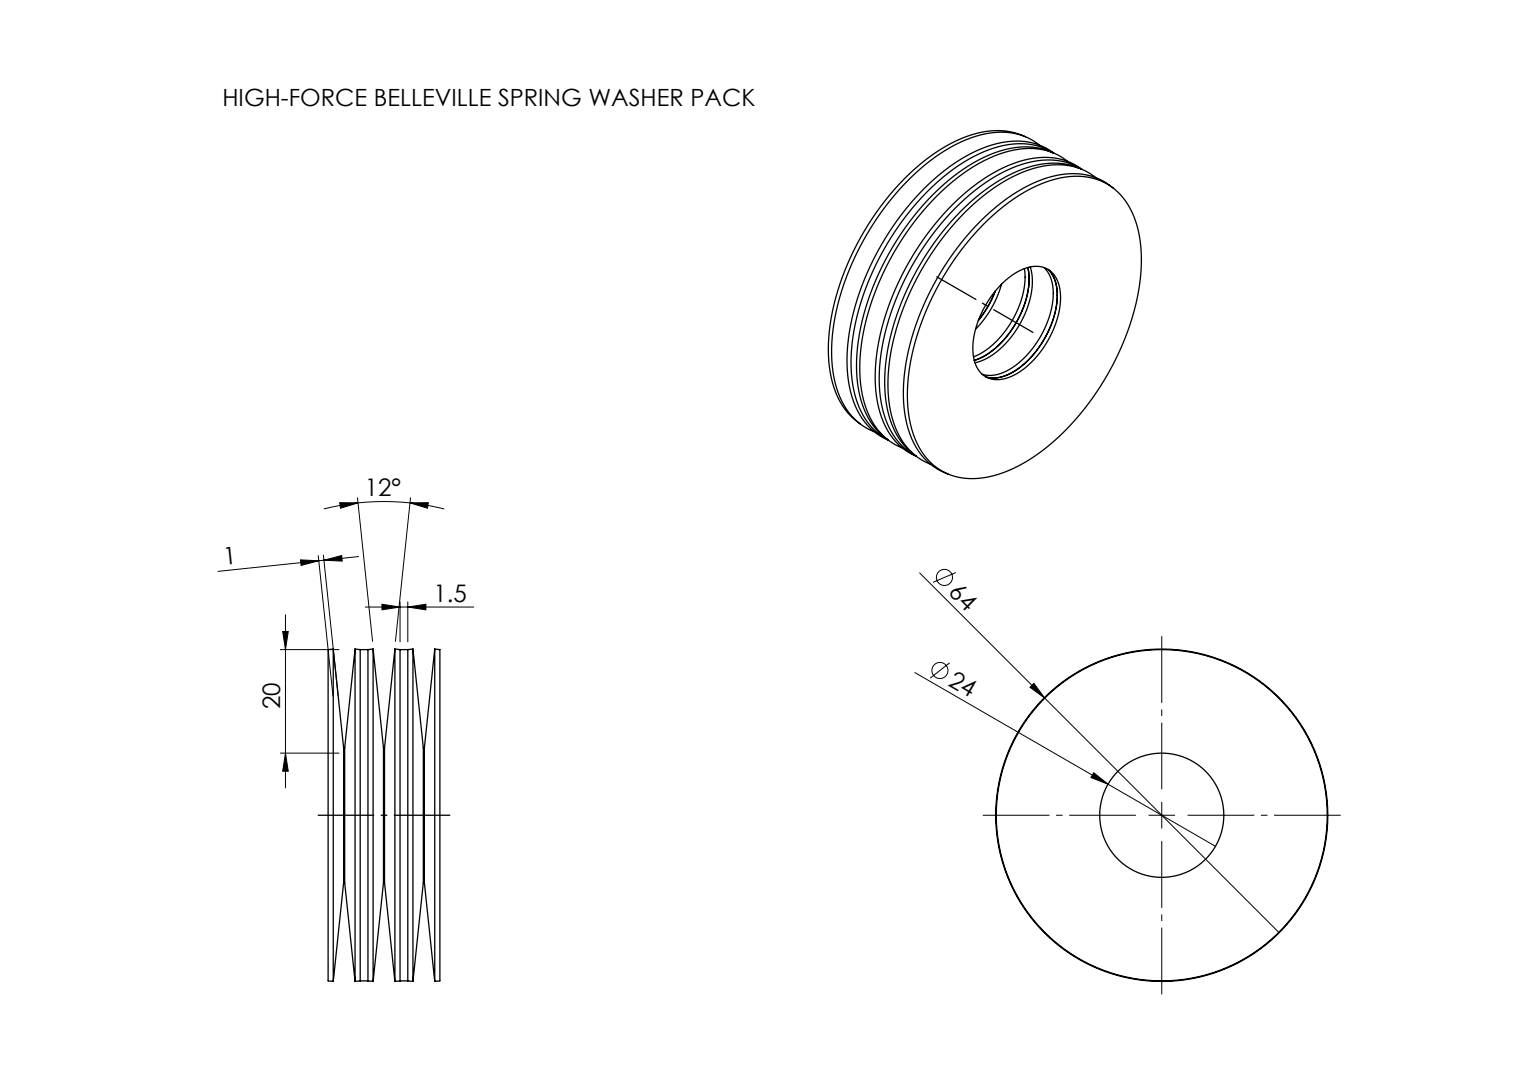
ISO-10303-21;
HEADER;
FILE_DESCRIPTION (('STEP AP214'),
    '1' );
FILE_NAME ('High-Force Belleville Spring Washer Pack.step',
    '2026-10-08T07:58:12',
    ( '' ),
    ( '' ),
    'SwSTEP 2.0',
    'SolidWorks 2026',
    '' );
FILE_SCHEMA (( 'AUTOMOTIVE_DESIGN' ));
ENDSEC;

DATA;
#82=VERTEX_POINT ( 'NONE', #32615 ) ;
#84=EDGE_LOOP ( 'NONE', ( #4042, #16247, #32529, #21714 ) ) ;
#116=ORIENTED_EDGE ( 'NONE', *, *, #1238, .F. ) ;
#123=ORIENTED_EDGE ( 'NONE', *, *, #8294, .T. ) ;
#126=CONICAL_SURFACE ( 'NONE', #19149, 32.00000000000005684, 0.1047197551196217685 ) ;
#134=CARTESIAN_POINT ( 'NONE',  ( 108.1100194822685836, 155.0000000000000000, 0.000000000000000000 ) ) ;
#174=( NAMED_UNIT ( * ) SI_UNIT ( $, .STERADIAN. ) SOLID_ANGLE_UNIT ( ) );
#179=EDGE_CURVE ( 'NONE', #29148, #5220, #18847, .T. ) ;
#189=CARTESIAN_POINT ( 'NONE',  ( 90.49452189536829394, 155.0000000000000000, 0.000000000000000000 ) ) ;
#195=CIRCLE ( 'NONE', #24668, 12.10452846326762177 ) ;
#196=CARTESIAN_POINT ( 'NONE',  ( 93.60208470531338776, 155.0000000000000000, 12.00000000000001066 ) ) ;
#210=VERTEX_POINT ( 'NONE', #17453 ) ;
#228=CIRCLE ( 'NONE', #27934, 13.00000000000001066 ) ;
#244=ORIENTED_EDGE ( 'NONE', *, *, #9158, .T. ) ;
#290=DIRECTION ( 'NONE',  ( 1.000000000000000000, -0.000000000000000000, -0.000000000000000000 ) ) ;
#316=DIRECTION ( 'NONE',  ( 0.000000000000000000, 0.000000000000000000, -1.000000000000000000 ) ) ;
#330=FILL_AREA_STYLE ('',( #26891 ) ) ;
#360=ORIENTED_EDGE ( 'NONE', *, *, #7714, .F. ) ;
#380=DIRECTION ( 'NONE',  ( -1.000000000000000000, 0.000000000000000000, 0.000000000000000000 ) ) ;
#424=DIRECTION ( 'NONE',  ( 0.000000000000000000, 0.000000000000000000, -1.000000000000000000 ) ) ;
#445=ADVANCED_FACE ( 'NONE', ( #32704 ), #17380, .F. ) ;
#456=VECTOR ( 'NONE', #17521, 1000.000000000000227 ) ;
#471=CIRCLE ( 'NONE', #10841, 12.10452846326762177 ) ;
#546=VERTEX_POINT ( 'NONE', #19601 ) ;
#555=LINE ( 'NONE', #10948, #13247 ) ;
#563=CARTESIAN_POINT ( 'NONE',  ( 102.4138169258850581, 155.0000000000000000, 0.000000000000000000 ) ) ;
#611=FACE_OUTER_BOUND ( 'NONE', #24311, .T. ) ;
#622=EDGE_CURVE ( 'NONE', #30802, #33225, #4723, .T. ) ;
#624=EDGE_CURVE ( 'NONE', #17270, #23382, #19967, .T. ) ;
#631=CARTESIAN_POINT ( 'NONE',  ( 100.2066581602377653, 155.0000000000000000, -13.00000000000001066 ) ) ;
#701=AXIS2_PLACEMENT_3D ( 'NONE', #11341, #16437, #6045 ) ;
#707=CARTESIAN_POINT ( 'NONE',  ( 94.70964751525852421, 155.0000000000000000, 32.10452846326766974 ) ) ;
#715=CIRCLE ( 'NONE', #5600, 13.00000000000003908 ) ;
#727=DIRECTION ( 'NONE',  ( 1.000000000000000000, -0.000000000000000000, -0.000000000000000000 ) ) ;
#732=DIRECTION ( 'NONE',  ( 0.000000000000000000, 0.000000000000000000, 1.000000000000000000 ) ) ;
#748=CARTESIAN_POINT ( 'NONE',  ( 100.4058500716420781, 155.0000000000000000, 0.000000000000000000 ) ) ;
#764=ADVANCED_FACE ( 'NONE', ( #27053 ), #13424, .T. ) ;
#767=EDGE_CURVE ( 'NONE', #31501, #25247, #11551, .T. ) ;
#794=CARTESIAN_POINT ( 'NONE',  ( 101.3062541159399075, 155.0000000000000000, -12.00000000000001066 ) ) ;
#824=DIRECTION ( 'NONE',  ( 1.000000000000000000, -0.000000000000000000, -0.000000000000000000 ) ) ;
#849=LINE ( 'NONE', #23689, #23558 ) ;
#881=CONICAL_SURFACE ( 'NONE', #18301, 31.00000000000000000, 1.466076571675255957 ) ;
#885=CARTESIAN_POINT ( 'NONE',  ( 92.70168066101555837, 155.0000000000000000, -13.00000000000003908 ) ) ;
#889=VERTEX_POINT ( 'NONE', #33000 ) ;
#899=ORIENTED_EDGE ( 'NONE', *, *, #32978, .F. ) ;
#910=ORIENTED_EDGE ( 'NONE', *, *, #16888, .T. ) ;
#916=APPLICATION_CONTEXT ( 'automotive_design' ) ;
#931=EDGE_LOOP ( 'NONE', ( #7883, #32623, #17410, #12258 ) ) ;
#954=CARTESIAN_POINT ( 'NONE',  ( 109.0104235265664272, 155.0000000000000000, -11.99999999999998224 ) ) ;
#978=EDGE_CURVE ( 'NONE', #23779, #33225, #14441, .T. ) ;
#984=EDGE_LOOP ( 'NONE', ( #28690, #5687, #6551, #10597 ) ) ;
#1046=CARTESIAN_POINT ( 'NONE',  ( 89.50000000000002842, 155.0000000000000000, 0.000000000000000000 ) ) ;
#1054=EDGE_CURVE ( 'NONE', #14849, #9110, #2180, .T. ) ;
#1085=ORIENTED_EDGE ( 'NONE', *, *, #22443, .T. ) ;
#1106=EDGE_LOOP ( 'NONE', ( #29137, #28238, #18476, #24027 ) ) ;
#1150=VECTOR ( 'NONE', #31313, 1000.000000000000000 ) ;
#1161=ORIENTED_EDGE ( 'NONE', *, *, #624, .T. ) ;
#1186=DIRECTION ( 'NONE',  ( -0.1045284632676468234, 1.217938055844715641E-16, -0.9945218953682740670 ) ) ;
#1204=CIRCLE ( 'NONE', #21871, 32.10452846326769816 ) ;
#1216=DIRECTION ( 'NONE',  ( -0.1045284632676468234, 1.217938055844715641E-16, -0.9945218953682740670 ) ) ;
#1225=LINE ( 'NONE', #11455, #20091 ) ;
#1236=VECTOR ( 'NONE', #1186, 1000.000000000000000 ) ;
#1238=EDGE_CURVE ( 'NONE', #29217, #23382, #10861, .T. ) ;
#1251=AXIS2_PLACEMENT_3D ( 'NONE', #4410, #33022, #24855 ) ;
#1255=CARTESIAN_POINT ( 'NONE',  ( 99.30625411593993590, 155.0000000000000000, 0.000000000000000000 ) ) ;
#1263=AXIS2_PLACEMENT_3D ( 'NONE', #30747, #23072, #15236 ) ;
#1285=( GEOMETRIC_REPRESENTATION_CONTEXT ( 3 ) GLOBAL_UNCERTAINTY_ASSIGNED_CONTEXT ( ( #28742 ) ) GLOBAL_UNIT_ASSIGNED_CONTEXT ( ( #21117, #12788, #28297 ) ) REPRESENTATION_CONTEXT ( 'NONE', 'WORKASPACE' ) );
#1300=LINE ( 'NONE', #25129, #6401 ) ;
#1393=CARTESIAN_POINT ( 'NONE',  ( 103.3032345859876102, 155.0000000000000000, 0.000000000000000000 ) ) ;
#1394=EDGE_CURVE ( 'NONE', #20431, #4805, #4178, .T. ) ;
#1411=EDGE_CURVE ( 'NONE', #11140, #8132, #1300, .T. ) ;
#1412=CARTESIAN_POINT ( 'NONE',  ( 109.0104235265664272, 155.0000000000000000, 0.000000000000000000 ) ) ;
#1482=CONICAL_SURFACE ( 'NONE', #33017, 31.00000000000000000, 1.466076571675244411 ) ;
#1485=CONICAL_SURFACE ( 'NONE', #10213, 32.00000000000002842, 0.1047197551196464710 ) ;
#1493=AXIS2_PLACEMENT_3D ( 'NONE', #20677, #28516, #8228 ) ;
#1518=AXIS2_PLACEMENT_3D ( 'NONE', #2238, #23684, #33580 ) ;
#1519=CARTESIAN_POINT ( 'NONE',  ( 97.20416941062678973, 155.0000000000000000, -32.00000000000000000 ) ) ;
#1564=DIRECTION ( 'NONE',  ( 0.000000000000000000, 0.000000000000000000, -1.000000000000000000 ) ) ;
#1566=EDGE_LOOP ( 'NONE', ( #30199, #32332, #23952, #6736 ) ) ;
#1576=CARTESIAN_POINT ( 'NONE',  ( 92.60208470531341618, 155.0000000000000000, 31.00000000000000000 ) ) ;
#1579=AXIS2_PLACEMENT_3D ( 'NONE', #10338, #33321, #5373 ) ;
#1590=DIRECTION ( 'NONE',  ( 1.000000000000000000, -0.000000000000000000, -0.000000000000000000 ) ) ;
#1605=CONICAL_SURFACE ( 'NONE', #3771, 31.00000000000000000, 1.466076571675244411 ) ;
#1612=DIRECTION ( 'NONE',  ( 0.000000000000000000, 0.000000000000000000, -1.000000000000000000 ) ) ;
#1617=EDGE_LOOP ( 'NONE', ( #31985, #3988, #7749, #18258 ) ) ;
#1622=ORIENTED_EDGE ( 'NONE', *, *, #19447, .F. ) ;
#1694=VERTEX_POINT ( 'NONE', #5033 ) ;
#1705=EDGE_LOOP ( 'NONE', ( #13701, #14443, #3420, #26950 ) ) ;
#1724=CARTESIAN_POINT ( 'NONE',  ( 108.0049454219347354, 155.0000000000000000, 0.000000000000000000 ) ) ;
#1753=ADVANCED_FACE ( 'NONE', ( #12697 ), #31102, .F. ) ;
#1778=CIRCLE ( 'NONE', #1251, 12.00000000000001066 ) ;
#1787=CONICAL_SURFACE ( 'NONE', #24631, 32.10452846326766974, 1.466076571675243523 ) ;
#1802=DIRECTION ( 'NONE',  ( 1.000000000000000000, -0.000000000000000000, -0.000000000000000000 ) ) ;
#1897=DIRECTION ( 'NONE',  ( 0.000000000000000000, 0.000000000000000000, 1.000000000000000000 ) ) ;
#1912=CARTESIAN_POINT ( 'NONE',  ( 100.4058500716420781, 155.0000000000000000, 0.000000000000000000 ) ) ;
#1918=DIRECTION ( 'NONE',  ( 0.000000000000000000, 0.000000000000000000, -1.000000000000000000 ) ) ;
#1975=DIRECTION ( 'NONE',  ( 1.000000000000000000, -0.000000000000000000, -0.000000000000000000 ) ) ;
#1993=DIRECTION ( 'NONE',  ( 0.000000000000000000, 0.000000000000000000, -1.000000000000000000 ) ) ;
#1996=ORIENTED_EDGE ( 'NONE', *, *, #12415, .T. ) ;
#2013=FACE_OUTER_BOUND ( 'NONE', #29654, .T. ) ;
#2018=APPLICATION_CONTEXT ( 'automotive_design' ) ;
#2030=VECTOR ( 'NONE', #31162, 999.9999999999998863 ) ;
#2040=EDGE_CURVE ( 'NONE', #21429, #17270, #21992, .T. ) ;
#2041=DIRECTION ( 'NONE',  ( 1.000000000000000000, -0.000000000000000000, -0.000000000000000000 ) ) ;
#2047=ADVANCED_FACE ( 'NONE', ( #16205 ), #18935, .T. ) ;
#2067=DIRECTION ( 'NONE',  ( 0.000000000000000000, 0.000000000000000000, -1.000000000000000000 ) ) ;
#2074=DIRECTION ( 'NONE',  ( 1.000000000000000000, -0.000000000000000000, -0.000000000000000000 ) ) ;
#2090=CIRCLE ( 'NONE', #13506, 12.10452846326765020 ) ;
#2092=ORIENTED_EDGE ( 'NONE', *, *, #32224, .T. ) ;
#2095=EDGE_CURVE ( 'NONE', #31583, #27125, #471, .T. ) ;
#2103=AXIS2_PLACEMENT_3D ( 'NONE', #21080, #17861, #5416 ) ;
#2126=DIRECTION ( 'NONE',  ( -1.000000000000000000, 0.000000000000000000, 0.000000000000000000 ) ) ;
#2131=VECTOR ( 'NONE', #9268, 1000.000000000000000 ) ;
#2168=CARTESIAN_POINT ( 'NONE',  ( 92.60208470531341618, 155.0000000000000000, -12.10452846326763598 ) ) ;
#2180=LINE ( 'NONE', #2696, #10740 ) ;
#2186=CARTESIAN_POINT ( 'NONE',  ( 92.60208470531341618, 155.0000000000000000, 0.000000000000000000 ) ) ;
#2209=DIRECTION ( 'NONE',  ( 1.000000000000000000, -0.000000000000000000, -0.000000000000000000 ) ) ;
#2210=VERTEX_POINT ( 'NONE', #25054 ) ;
#2238=CARTESIAN_POINT ( 'NONE',  ( 97.20416941062678973, 155.0000000000000000, 0.000000000000000000 ) ) ;
#2248=DIRECTION ( 'NONE',  ( 0.000000000000000000, 0.000000000000000000, -1.000000000000000000 ) ) ;
#2284=AXIS2_PLACEMENT_3D ( 'NONE', #19617, #14669, #2067 ) ;
#2288=LINE ( 'NONE', #12842, #12668 ) ;
#2313=VECTOR ( 'NONE', #14414, 1000.000000000000114 ) ;
#2325=EDGE_CURVE ( 'NONE', #33225, #30802, #15185, .T. ) ;
#2357=DIRECTION ( 'NONE',  ( 1.000000000000000000, -0.000000000000000000, -0.000000000000000000 ) ) ;
#2368=AXIS2_PLACEMENT_3D ( 'NONE', #10280, #31377, #20658 ) ;
#2384=ORIENTED_EDGE ( 'NONE', *, *, #27422, .T. ) ;
#2397=CARTESIAN_POINT ( 'NONE',  ( 92.60208470531341618, 155.0000000000000000, 32.00000000000002842 ) ) ;
#2404=AXIS2_PLACEMENT_3D ( 'NONE', #8872, #11941, #4266 ) ;
#2457=ORIENTED_EDGE ( 'NONE', *, *, #7239, .F. ) ;
#2463=ORIENTED_EDGE ( 'NONE', *, *, #19799, .F. ) ;
#2483=DIRECTION ( 'NONE',  ( 0.000000000000000000, 0.000000000000000000, -1.000000000000000000 ) ) ;
#2490=CARTESIAN_POINT ( 'NONE',  ( 95.70416941062676131, 155.0000000000000000, 0.000000000000000000 ) ) ;
#2495=FACE_OUTER_BOUND ( 'NONE', #5360, .T. ) ;
#2548=CIRCLE ( 'NONE', #16678, 12.00000000000001066 ) ;
#2652=LINE ( 'NONE', #25643, #15958 ) ;
#2659=CARTESIAN_POINT ( 'NONE',  ( 92.60208470531341618, 155.0000000000000000, 12.10452846326765020 ) ) ;
#2696=CARTESIAN_POINT ( 'NONE',  ( 92.60208470531341618, 155.0000000000000000, -12.99999999999999822 ) ) ;
#2730=EDGE_CURVE ( 'NONE', #20904, #29148, #11559, .T. ) ;
#2735=EDGE_CURVE ( 'NONE', #20904, #6439, #27778, .T. ) ;
#2760=VERTEX_POINT ( 'NONE', #11222 ) ;
#2850=DIRECTION ( 'NONE',  ( 1.000000000000000000, -0.000000000000000000, -0.000000000000000000 ) ) ;
#2853=ADVANCED_FACE ( 'NONE', ( #21776 ), #30510, .T. ) ;
#2878=DIRECTION ( 'NONE',  ( 1.000000000000000000, -0.000000000000000000, -0.000000000000000000 ) ) ;
#2879=ORIENTED_EDGE ( 'NONE', *, *, #30577, .F. ) ;
#2942=DIRECTION ( 'NONE',  ( -0.1045284632676468234, 0.000000000000000000, 0.9945218953682740670 ) ) ;
#2962=CARTESIAN_POINT ( 'NONE',  ( 97.30927364589244632, 155.0000000000000000, 0.000000000000000000 ) ) ;
#2963=ORIENTED_EDGE ( 'NONE', *, *, #18143, .F. ) ;
#3002=ORIENTED_EDGE ( 'NONE', *, *, #15223, .F. ) ;
#3028=ADVANCED_FACE ( 'NONE', ( #2013 ), #6784, .F. ) ;
#3080=AXIS2_PLACEMENT_3D ( 'NONE', #20994, #31391, #8061 ) ;
#3117=LINE ( 'NONE', #30021, #19378 ) ;
#3146=VECTOR ( 'NONE', #32555, 1000.000000000000000 ) ;
#3149=EDGE_LOOP ( 'NONE', ( #21685, #21772, #23410, #22654 ) ) ;
#3154=DIRECTION ( 'NONE',  ( 1.000000000000000000, -0.000000000000000000, -0.000000000000000000 ) ) ;
#3157=VERTEX_POINT ( 'NONE', #27733 ) ;
#3188=CARTESIAN_POINT ( 'NONE',  ( 98.19869130599479945, 155.0000000000000000, -32.10452846326769816 ) ) ;
#3207=ORIENTED_EDGE ( 'NONE', *, *, #767, .T. ) ;
#3259=CARTESIAN_POINT ( 'NONE',  ( 92.60208470531341618, 155.0000000000000000, 0.000000000000000000 ) ) ;
#3279=ADVANCED_FACE ( 'NONE', ( #4905 ), #25518, .T. ) ;
#3308=DIRECTION ( 'NONE',  ( -0.9945218953682772867, 1.280104479604772081E-17, -0.1045284632676156678 ) ) ;
#3316=CARTESIAN_POINT ( 'NONE',  ( 100.4058500716420781, 155.0000000000000000, -12.99999999999998401 ) ) ;
#3346=FACE_OUTER_BOUND ( 'NONE', #29316, .T. ) ;
#3358=CONICAL_SURFACE ( 'NONE', #11467, 32.10452846326769816, 1.466076571675243523 ) ;
#3415=VECTOR ( 'NONE', #9617, 1000.000000000000000 ) ;
#3420=ORIENTED_EDGE ( 'NONE', *, *, #23975, .T. ) ;
#3440=CARTESIAN_POINT ( 'NONE',  ( 100.2066581602377653, 155.0000000000000000, 0.000000000000000000 ) ) ;
#3445=EDGE_CURVE ( 'NONE', #889, #23658, #5075, .T. ) ;
#3446=VECTOR ( 'NONE', #9745, 1000.000000000000000 ) ;
#3479=CARTESIAN_POINT ( 'NONE',  ( 92.60208470531341618, 155.0000000000000000, -31.00000000000000000 ) ) ;
#3490=AXIS2_PLACEMENT_3D ( 'NONE', #3890, #6624, #19900 ) ;
#3537=EDGE_CURVE ( 'NONE', #20010, #29148, #19314, .T. ) ;
#3619=ORIENTED_EDGE ( 'NONE', *, *, #23140, .T. ) ;
#3621=AXIS2_PLACEMENT_3D ( 'NONE', #11749, #27088, #9530 ) ;
#3627=DIRECTION ( 'NONE',  ( 0.000000000000000000, 0.000000000000000000, 1.000000000000000000 ) ) ;
#3650=FACE_OUTER_BOUND ( 'NONE', #25283, .T. ) ;
#3652=ORIENTED_EDGE ( 'NONE', *, *, #30577, .T. ) ;
#3660=ORIENTED_EDGE ( 'NONE', *, *, #2325, .T. ) ;
#3661=LINE ( 'NONE', #7590, #25185 ) ;
#3665=CONICAL_SURFACE ( 'NONE', #8043, 31.00000000000000000, 1.466076571675243967 ) ;
#3667=CIRCLE ( 'NONE', #23258, 31.00000000000000000 ) ;
#3670=DIRECTION ( 'NONE',  ( 0.000000000000000000, 0.000000000000000000, -1.000000000000000000 ) ) ;
#3694=VECTOR ( 'NONE', #17304, 1000.000000000000227 ) ;
#3713=CARTESIAN_POINT ( 'NONE',  ( 107.0104235265664556, 155.0000000000000000, -11.99999999999998224 ) ) ;
#3715=DIRECTION ( 'NONE',  ( 0.000000000000000000, 0.000000000000000000, -1.000000000000000000 ) ) ;
#3744=ORIENTED_EDGE ( 'NONE', *, *, #8275, .T. ) ;
#3753=VECTOR ( 'NONE', #32543, 1000.000000000000000 ) ;
#3771=AXIS2_PLACEMENT_3D ( 'NONE', #1393, #29678, #11783 ) ;
#3778=DIRECTION ( 'NONE',  ( 1.000000000000000000, -0.000000000000000000, -0.000000000000000000 ) ) ;
#3786=EDGE_LOOP ( 'NONE', ( #21693, #360, #32034, #18428 ) ) ;
#3805=ORIENTED_EDGE ( 'NONE', *, *, #29067, .T. ) ;
#3869=EDGE_LOOP ( 'NONE', ( #22538, #19080, #7962, #23492 ) ) ;
#3881=CARTESIAN_POINT ( 'NONE',  ( 105.0134430565187387, 155.0000000000000000, 0.000000000000000000 ) ) ;
#3890=CARTESIAN_POINT ( 'NONE',  ( 95.59906517536109050, 155.0000000000000000, 0.000000000000000000 ) ) ;
#3903=ORIENTED_EDGE ( 'NONE', *, *, #15621, .F. ) ;
#3925=CIRCLE ( 'NONE', #14822, 31.00000000000000000 ) ;
#3952=CIRCLE ( 'NONE', #23003, 13.00000000000003908 ) ;
#3977=AXIS2_PLACEMENT_3D ( 'NONE', #10455, #380, #25940 ) ;
#3982=DIRECTION ( 'NONE',  ( 1.000000000000000000, -0.000000000000000000, -0.000000000000000000 ) ) ;
#3988=ORIENTED_EDGE ( 'NONE', *, *, #4099, .T. ) ;
#4004=AXIS2_PLACEMENT_3D ( 'NONE', #13608, #6100, #18734 ) ;
#4006=DIRECTION ( 'NONE',  ( 0.000000000000000000, 0.000000000000000000, -1.000000000000000000 ) ) ;
#4042=ORIENTED_EDGE ( 'NONE', *, *, #11060, .F. ) ;
#4049=AXIS2_PLACEMENT_3D ( 'NONE', #21081, #18855, #13739 ) ;
#4058=EDGE_CURVE ( 'NONE', #19467, #20904, #8066, .T. ) ;
#4093=CARTESIAN_POINT ( 'NONE',  ( 89.50000000000002842, 155.0000000000000000, 32.00000000000002842 ) ) ;
#4099=EDGE_CURVE ( 'NONE', #26344, #8252, #7568, .T. ) ;
#4131=CARTESIAN_POINT ( 'NONE',  ( 93.60208470531338776, 155.0000000000000000, 0.000000000000000000 ) ) ;
#4154=CARTESIAN_POINT ( 'NONE',  ( 97.30927364589244632, 155.0000000000000000, -31.00000000000000000 ) ) ;
#4168=CARTESIAN_POINT ( 'NONE',  ( 92.59660660068168170, 155.0000000000000000, 12.10452846326765020 ) ) ;
#4178=LINE ( 'NONE', #32796, #3694 ) ;
#4179=AXIS2_PLACEMENT_3D ( 'NONE', #4929, #9701, #31009 ) ;
#4205=AXIS2_PLACEMENT_3D ( 'NONE', #7733, #15048, #23060 ) ;
#4209=EDGE_LOOP ( 'NONE', ( #7500, #7245, #27184, #2457 ) ) ;
#4216=DIRECTION ( 'NONE',  ( 0.000000000000000000, 0.000000000000000000, -1.000000000000000000 ) ) ;
#4219=DIRECTION ( 'NONE',  ( 1.000000000000000000, -0.000000000000000000, -0.000000000000000000 ) ) ;
#4253=AXIS2_PLACEMENT_3D ( 'NONE', #31822, #23662, #13429 ) ;
#4266=DIRECTION ( 'NONE',  ( 1.000000000000000000, 0.000000000000000000, 0.000000000000000000 ) ) ;
#4271=SURFACE_STYLE_FILL_AREA ( #27603 ) ;
#4277=ADVANCED_FACE ( 'NONE', ( #28344 ), #8784, .F. ) ;
#4280=CARTESIAN_POINT ( 'NONE',  ( 110.1179863365115636, 155.0000000000000000, -32.10452846326764131 ) ) ;
#4283=VECTOR ( 'NONE', #28740, 1000.000000000000114 ) ;
#4291=CARTESIAN_POINT ( 'NONE',  ( 98.19869130599479945, 155.0000000000000000, 32.10452846326769816 ) ) ;
#4293=CYLINDRICAL_SURFACE ( 'NONE', #33547, 12.99999999999999822 ) ;
#4304=CIRCLE ( 'NONE', #27694, 12.00000000000001066 ) ;
#4310=CARTESIAN_POINT ( 'NONE',  ( 95.59906517536109050, 155.0000000000000000, 31.00000000000000000 ) ) ;
#4327=VERTEX_POINT ( 'NONE', #8720 ) ;
#4334=ORIENTED_EDGE ( 'NONE', *, *, #32696, .F. ) ;
#4340=DIRECTION ( 'NONE',  ( 0.000000000000000000, 0.000000000000000000, -1.000000000000000000 ) ) ;
#4342=EDGE_CURVE ( 'NONE', #26926, #8252, #19662, .T. ) ;
#4350=CARTESIAN_POINT ( 'NONE',  ( 92.60208470531341618, 155.0000000000000000, 0.000000000000000000 ) ) ;
#4354=EDGE_CURVE ( 'NONE', #3157, #20526, #13668, .T. ) ;
#4377=CARTESIAN_POINT ( 'NONE',  ( 89.50000000000002842, 155.0000000000000000, 0.000000000000000000 ) ) ;
#4396=EDGE_CURVE ( 'NONE', #29530, #21869, #24392, .T. ) ;
#4410=CARTESIAN_POINT ( 'NONE',  ( 101.3062541159399075, 155.0000000000000000, 0.000000000000000000 ) ) ;
#4422=ORIENTED_EDGE ( 'NONE', *, *, #13855, .T. ) ;
#4431=EDGE_LOOP ( 'NONE', ( #20479, #3207, #22862, #15414 ) ) ;
#4433=DIRECTION ( 'NONE',  ( 0.000000000000000000, 0.000000000000000000, -1.000000000000000000 ) ) ;
#4442=AXIS2_PLACEMENT_3D ( 'NONE', #15260, #7433, #28384 ) ;
#4466=DIRECTION ( 'NONE',  ( 1.000000000000000000, -0.000000000000000000, -0.000000000000000000 ) ) ;
#4500=EDGE_LOOP ( 'NONE', ( #6558, #20766, #11342, #4422 ) ) ;
#4511=DIRECTION ( 'NONE',  ( 0.000000000000000000, 0.000000000000000000, -1.000000000000000000 ) ) ;
#4540=EDGE_CURVE ( 'NONE', #2760, #23658, #27296, .T. ) ;
#4550=AXIS2_PLACEMENT_3D ( 'NONE', #2962, #24060, #732 ) ;
#4568=COLOUR_RGB ( '', 0.09019608, 0.27058824, 0.51372549) ;
#4601=ORIENTED_EDGE ( 'NONE', *, *, #6376, .F. ) ;
#4603=DIRECTION ( 'NONE',  ( 1.000000000000000000, -0.000000000000000000, -0.000000000000000000 ) ) ;
#4613=CARTESIAN_POINT ( 'NONE',  ( 110.1179863365115636, 155.0000000000000000, 0.000000000000000000 ) ) ;
#4664=CARTESIAN_POINT ( 'NONE',  ( 105.9028607166213192, 155.0000000000000000, -32.10452846326769816 ) ) ;
#4685=ADVANCED_FACE ( 'NONE', ( #9555 ), #3358, .T. ) ;
#4712=LINE ( 'NONE', #2168, #24875 ) ;
#4723=CIRCLE ( 'NONE', #6345, 31.00000000000000000 ) ;
#4805=VERTEX_POINT ( 'NONE', #30513 ) ;
#4830=DIRECTION ( 'NONE',  ( -1.000000000000000000, 0.000000000000000000, 0.000000000000000000 ) ) ;
#4856=AXIS2_PLACEMENT_3D ( 'NONE', #1255, #1590, #9257 ) ;
#4887=DIRECTION ( 'NONE',  ( 0.000000000000000000, 0.000000000000000000, -1.000000000000000000 ) ) ;
#4905=FACE_OUTER_BOUND ( 'NONE', #8529, .T. ) ;
#4929=CARTESIAN_POINT ( 'NONE',  ( 91.60208470531341618, 155.0000000000000000, 0.000000000000000000 ) ) ;
#4988=ORIENTED_EDGE ( 'NONE', *, *, #26148, .T. ) ;
#5033=CARTESIAN_POINT ( 'NONE',  ( 100.3007760113082156, 155.0000000000000000, 12.10452846326762177 ) ) ;
#5037=CARTESIAN_POINT ( 'NONE',  ( 92.60208470531341618, 155.0000000000000000, 0.000000000000000000 ) ) ;
#5051=CARTESIAN_POINT ( 'NONE',  ( 95.70416941062676131, 155.0000000000000000, 0.000000000000000000 ) ) ;
#5071=AXIS2_PLACEMENT_3D ( 'NONE', #23018, #33416, #10090 ) ;
#5072=DIRECTION ( 'NONE',  ( 1.000000000000000000, -0.000000000000000000, -0.000000000000000000 ) ) ;
#5075=LINE ( 'NONE', #20416, #29977 ) ;
#5079=CARTESIAN_POINT ( 'NONE',  ( 107.0104235265664556, 155.0000000000000000, 0.000000000000000000 ) ) ;
#5085=CIRCLE ( 'NONE', #33395, 32.10452846326766974 ) ;
#5088=AXIS2_PLACEMENT_3D ( 'NONE', #1412, #30031, #6696 ) ;
#5099=AXIS2_PLACEMENT_3D ( 'NONE', #7320, #7822, #20756 ) ;
#5106=ORIENTED_EDGE ( 'NONE', *, *, #14915, .T. ) ;
#5144=ORIENTED_EDGE ( 'NONE', *, *, #28298, .T. ) ;
#5201=ADVANCED_FACE ( 'NONE', ( #19068 ), #26631, .T. ) ;
#5204=DIRECTION ( 'NONE',  ( 0.000000000000000000, 0.000000000000000000, -1.000000000000000000 ) ) ;
#5220=VERTEX_POINT ( 'NONE', #11569 ) ;
#5245=CARTESIAN_POINT ( 'NONE',  ( 111.1125082318798007, 155.0000000000000000, -32.00000000000002842 ) ) ;
#5246=CYLINDRICAL_SURFACE ( 'NONE', #17117, 32.00000000000002842 ) ;
#5264=ORIENTED_EDGE ( 'NONE', *, *, #7911, .F. ) ;
#5274=CARTESIAN_POINT ( 'NONE',  ( 105.0134430565187387, 155.0000000000000000, 0.000000000000000000 ) ) ;
#5281=LINE ( 'NONE', #18239, #15726 ) ;
#5282=AXIS2_PLACEMENT_3D ( 'NONE', #28932, #2878, #316 ) ;
#5284=AXIS2_PLACEMENT_3D ( 'NONE', #25891, #28451, #26066 ) ;
#5287=CARTESIAN_POINT ( 'NONE',  ( 105.0134430565187387, 155.0000000000000000, -31.00000000000000000 ) ) ;
#5290=DIRECTION ( 'NONE',  ( -1.000000000000000000, 0.000000000000000000, 0.000000000000000000 ) ) ;
#5295=DIRECTION ( 'NONE',  ( 0.000000000000000000, 0.000000000000000000, -1.000000000000000000 ) ) ;
#5355=CONICAL_SURFACE ( 'NONE', #29307, 11.99999999999998224, 0.1047197551197030924 ) ;
#5360=EDGE_LOOP ( 'NONE', ( #22959, #5605, #26874, #27254 ) ) ;
#5373=DIRECTION ( 'NONE',  ( 0.000000000000000000, 0.000000000000000000, -1.000000000000000000 ) ) ;
#5378=AXIS2_PLACEMENT_3D ( 'NONE', #563, #727, #13838 ) ;
#5381=DIRECTION ( 'NONE',  ( 0.000000000000000000, 0.000000000000000000, -1.000000000000000000 ) ) ;
#5407=ORIENTED_EDGE ( 'NONE', *, *, #20406, .T. ) ;
#5416=DIRECTION ( 'NONE',  ( 0.000000000000000000, 0.000000000000000000, -1.000000000000000000 ) ) ;
#5417=FACE_OUTER_BOUND ( 'NONE', #16351, .T. ) ;
#5486=DIRECTION ( 'NONE',  ( 0.000000000000000000, 0.000000000000000000, 1.000000000000000000 ) ) ;
#5490=DIRECTION ( 'NONE',  ( 1.000000000000000000, -0.000000000000000000, -0.000000000000000000 ) ) ;
#5520=DIRECTION ( 'NONE',  ( 1.000000000000000000, -0.000000000000000000, -0.000000000000000000 ) ) ;
#5559=VECTOR ( 'NONE', #10869, 1000.000000000000000 ) ;
#5565=LINE ( 'NONE', #794, #7813 ) ;
#5595=ORIENTED_EDGE ( 'NONE', *, *, #6177, .T. ) ;
#5600=AXIS2_PLACEMENT_3D ( 'NONE', #28909, #8299, #29080 ) ;
#5605=ORIENTED_EDGE ( 'NONE', *, *, #12415, .F. ) ;
#5608=SURFACE_SIDE_STYLE ('',( #28950 ) ) ;
#5662=CARTESIAN_POINT ( 'NONE',  ( 89.50000000000002842, 155.0000000000000000, 32.00000000000002842 ) ) ;
#5687=ORIENTED_EDGE ( 'NONE', *, *, #25979, .T. ) ;
#5710=DIRECTION ( 'NONE',  ( 1.000000000000000000, -0.000000000000000000, -0.000000000000000000 ) ) ;
#5726=DIRECTION ( 'NONE',  ( -0.9945218953682717355, 1.280104479605409178E-17, -0.1045284632676676817 ) ) ;
#5733=DIRECTION ( 'NONE',  ( 1.000000000000000000, -0.000000000000000000, -0.000000000000000000 ) ) ;
#5809=CARTESIAN_POINT ( 'NONE',  ( 92.60208470531341618, 155.0000000000000000, 12.10452846326766441 ) ) ;
#5816=CIRCLE ( 'NONE', #16147, 12.00000000000001066 ) ;
#5849=DIRECTION ( 'NONE',  ( 0.000000000000000000, 0.000000000000000000, -1.000000000000000000 ) ) ;
#5850=VECTOR ( 'NONE', #31344, 1000.000000000000000 ) ;
#5861=ORIENTED_EDGE ( 'NONE', *, *, #8546, .T. ) ;
#5878=AXIS2_PLACEMENT_3D ( 'NONE', #21765, #824, #31663 ) ;
#5884=ORIENTED_EDGE ( 'NONE', *, *, #9752, .T. ) ;
#5968=ORIENTED_EDGE ( 'NONE', *, *, #10643, .F. ) ;
#5977=CARTESIAN_POINT ( 'NONE',  ( 92.60208470531341618, 155.0000000000000000, 0.000000000000000000 ) ) ;
#5978=DIRECTION ( 'NONE',  ( 1.000000000000000000, -0.000000000000000000, -0.000000000000000000 ) ) ;
#5994=ADVANCED_FACE ( 'NONE', ( #10816 ), #6957, .F. ) ;
#6014=ORIENTED_EDGE ( 'NONE', *, *, #18714, .T. ) ;
#6045=DIRECTION ( 'NONE',  ( 0.000000000000000000, 0.000000000000000000, 1.000000000000000000 ) ) ;
#6063=DIRECTION ( 'NONE',  ( 0.000000000000000000, 0.000000000000000000, -1.000000000000000000 ) ) ;
#6081=CIRCLE ( 'NONE', #4442, 31.00000000000000000 ) ;
#6087=DIRECTION ( 'NONE',  ( 1.000000000000000000, -0.000000000000000000, -0.000000000000000000 ) ) ;
#6100=DIRECTION ( 'NONE',  ( 1.000000000000000000, -0.000000000000000000, -0.000000000000000000 ) ) ;
#6144=CYLINDRICAL_SURFACE ( 'NONE', #21582, 13.00000000000002487 ) ;
#6177=EDGE_CURVE ( 'NONE', #26453, #17290, #17884, .T. ) ;
#6236=ADVANCED_FACE ( 'NONE', ( #24242 ), #5355, .F. ) ;
#6293=LINE ( 'NONE', #24531, #1236 ) ;
#6337=DIRECTION ( 'NONE',  ( 1.000000000000000000, -0.000000000000000000, -0.000000000000000000 ) ) ;
#6345=AXIS2_PLACEMENT_3D ( 'NONE', #17892, #15161, #25554 ) ;
#6376=EDGE_CURVE ( 'NONE', #33389, #20431, #32554, .T. ) ;
#6401=VECTOR ( 'NONE', #11857, 1000.000000000000000 ) ;
#6403=CONICAL_SURFACE ( 'NONE', #4856, 12.00000000000001066, 0.1047197551196174109 ) ;
#6430=EDGE_CURVE ( 'NONE', #20010, #25373, #16775, .T. ) ;
#6439=VERTEX_POINT ( 'NONE', #5245 ) ;
#6458=AXIS2_PLACEMENT_3D ( 'NONE', #7613, #12878, #10343 ) ;
#6472=ORIENTED_EDGE ( 'NONE', *, *, #13635, .T. ) ;
#6507=DIRECTION ( 'NONE',  ( 1.000000000000000000, -0.000000000000000000, -0.000000000000000000 ) ) ;
#6518=ORIENTED_EDGE ( 'NONE', *, *, #9752, .F. ) ;
#6528=CARTESIAN_POINT ( 'NONE',  ( 107.9108275708642850, 155.0000000000000000, 13.00000000000001066 ) ) ;
#6549=DIRECTION ( 'NONE',  ( 1.000000000000000000, -0.000000000000000000, -0.000000000000000000 ) ) ;
#6551=ORIENTED_EDGE ( 'NONE', *, *, #32978, .T. ) ;
#6558=ORIENTED_EDGE ( 'NONE', *, *, #26437, .F. ) ;
#6563=ORIENTED_EDGE ( 'NONE', *, *, #25009, .T. ) ;
#6610=EDGE_LOOP ( 'NONE', ( #4334, #910, #23987, #29946 ) ) ;
#6613=DIRECTION ( 'NONE',  ( 0.000000000000000000, 0.000000000000000000, -1.000000000000000000 ) ) ;
#6624=DIRECTION ( 'NONE',  ( 1.000000000000000000, -0.000000000000000000, -0.000000000000000000 ) ) ;
#6645=ORIENTED_EDGE ( 'NONE', *, *, #3445, .T. ) ;
#6655=DIRECTION ( 'NONE',  ( 1.000000000000000000, -0.000000000000000000, -0.000000000000000000 ) ) ;
#6659=CIRCLE ( 'NONE', #25707, 12.10452846326765020 ) ;
#6696=DIRECTION ( 'NONE',  ( 0.000000000000000000, 0.000000000000000000, -1.000000000000000000 ) ) ;
#6708=AXIS2_PLACEMENT_3D ( 'NONE', #12654, #30215, #20496 ) ;
#6715=AXIS2_PLACEMENT_3D ( 'NONE', #19469, #24586, #29070 ) ;
#6718=ORIENTED_EDGE ( 'NONE', *, *, #30798, .T. ) ;
#6736=ORIENTED_EDGE ( 'NONE', *, *, #22443, .F. ) ;
#6784=CYLINDRICAL_SURFACE ( 'NONE', #20710, 12.10452846326766441 ) ;
#6809=DIRECTION ( 'NONE',  ( 1.000000000000000000, -0.000000000000000000, -0.000000000000000000 ) ) ;
#6823=ORIENTED_EDGE ( 'NONE', *, *, #14588, .T. ) ;
#6854=ADVANCED_FACE ( 'NONE', ( #7092 ), #30381, .F. ) ;
#6889=CLOSED_SHELL ( 'NONE', ( #16015, #28692, #23967, #764, #22279, #20964, #21242, #32054, #22481, #16585, #26023, #2047, #23326, #4685, #3279, #5201, #29139, #4277, #6236, #3028, #24156, #9967, #445, #8141, #18499, #21885, #30768, #16053, #10412, #6854, #11378, #16941, #25587, #14513, #14358, #23296, #25356, #18137, #5994, #27182, #21473, #24496, #23342, #28496, #9123, #1753, #10464, #28128, #24367, #13139, #32828, #2853, #31257, #9493, #29920, #17866, #14478, #13898, #6901, #17085, #27664, #32558, #13294, #14774, #13459, #26384, #15813, #23871 ) ) ;
#6901=ADVANCED_FACE ( 'NONE', ( #30770 ), #12456, .T. ) ;
#6906=CARTESIAN_POINT ( 'NONE',  ( 93.60208470531338776, 155.0000000000000000, 12.00000000000001066 ) ) ;
#6934=CONICAL_SURFACE ( 'NONE', #29795, 11.99999999999998224, 0.1047197551196726167 ) ;
#6944=AXIS2_PLACEMENT_3D ( 'NONE', #29705, #21865, #32597 ) ;
#6953=SHAPE_REPRESENTATION_RELATIONSHIP ( 'NONE' , 'NONE' ,  #17605, #9595 ) ;
#6957=CONICAL_SURFACE ( 'NONE', #26006, 31.00000000000000000, 1.466076571675244411 ) ;
#6991=VERTEX_POINT ( 'NONE', #20882 ) ;
#7034=VECTOR ( 'NONE', #21206, 1000.000000000000000 ) ;
#7076=FACE_OUTER_BOUND ( 'NONE', #3786, .T. ) ;
#7089=EDGE_CURVE ( 'NONE', #23658, #2760, #17368, .T. ) ;
#7092=FACE_OUTER_BOUND ( 'NONE', #30878, .T. ) ;
#7141=LINE ( 'NONE', #1519, #29532 ) ;
#7198=CARTESIAN_POINT ( 'NONE',  ( 109.0104235265664272, 155.0000000000000000, 11.99999999999998224 ) ) ;
#7226=AXIS2_PLACEMENT_3D ( 'NONE', #2490, #17990, #5204 ) ;
#7239=EDGE_CURVE ( 'NONE', #30802, #12687, #26815, .T. ) ;
#7242=ORIENTED_EDGE ( 'NONE', *, *, #12909, .T. ) ;
#7245=ORIENTED_EDGE ( 'NONE', *, *, #19318, .T. ) ;
#7251=AXIS2_PLACEMENT_3D ( 'NONE', #30025, #19462, #14511 ) ;
#7284=DIRECTION ( 'NONE',  ( 1.000000000000000000, -0.000000000000000000, -0.000000000000000000 ) ) ;
#7292=EDGE_CURVE ( 'NONE', #6439, #5220, #8932, .T. ) ;
#7320=CARTESIAN_POINT ( 'NONE',  ( 92.50248874961125978, 155.0000000000000000, 0.000000000000000000 ) ) ;
#7321=( GEOMETRIC_REPRESENTATION_CONTEXT ( 3 ) GLOBAL_UNCERTAINTY_ASSIGNED_CONTEXT ( ( #15858 ) ) GLOBAL_UNIT_ASSIGNED_CONTEXT ( ( #32334, #9332, #29956 ) ) REPRESENTATION_CONTEXT ( 'NONE', 'WORKASPACE' ) );
#7367=FACE_OUTER_BOUND ( 'NONE', #31700, .T. ) ;
#7420=CARTESIAN_POINT ( 'NONE',  ( 107.0104235265664556, 155.0000000000000000, 11.99999999999998224 ) ) ;
#7423=DIRECTION ( 'NONE',  ( 1.000000000000000000, -0.000000000000000000, -0.000000000000000000 ) ) ;
#7429=EDGE_CURVE ( 'NONE', #17208, #10473, #32767, .T. ) ;
#7433=DIRECTION ( 'NONE',  ( 1.000000000000000000, -0.000000000000000000, -0.000000000000000000 ) ) ;
#7497=AXIS2_PLACEMENT_3D ( 'NONE', #17104, #4830, #12661 ) ;
#7500=ORIENTED_EDGE ( 'NONE', *, *, #2325, .F. ) ;
#7568=LINE ( 'NONE', #5662, #18598 ) ;
#7590=CARTESIAN_POINT ( 'NONE',  ( 92.60208470531341618, 155.0000000000000000, 13.00000000000002487 ) ) ;
#7613=CARTESIAN_POINT ( 'NONE',  ( 105.9028607166213192, 155.0000000000000000, 0.000000000000000000 ) ) ;
#7698=DIRECTION ( 'NONE',  ( -0.9945218953682714025, 0.000000000000000000, 0.1045284632676720116 ) ) ;
#7705=CARTESIAN_POINT ( 'NONE',  ( 95.59906517536109050, 155.0000000000000000, -31.00000000000000000 ) ) ;
#7714=EDGE_CURVE ( 'NONE', #21804, #19123, #4304, .T. ) ;
#7715=EDGE_CURVE ( 'NONE', #10473, #546, #21711, .T. ) ;
#7733=CARTESIAN_POINT ( 'NONE',  ( 92.60208470531341618, 155.0000000000000000, 0.000000000000000000 ) ) ;
#7745=CONICAL_SURFACE ( 'NONE', #8788, 32.00000000000002842, 0.1047197551196784177 ) ;
#7749=ORIENTED_EDGE ( 'NONE', *, *, #4342, .F. ) ;
#7797=CARTESIAN_POINT ( 'NONE',  ( 92.60208470531341618, 155.0000000000000000, 0.000000000000000000 ) ) ;
#7813=VECTOR ( 'NONE', #5726, 1000.000000000000114 ) ;
#7822=DIRECTION ( 'NONE',  ( 1.000000000000000000, -0.000000000000000000, -0.000000000000000000 ) ) ;
#7883=ORIENTED_EDGE ( 'NONE', *, *, #18291, .F. ) ;
#7911=EDGE_CURVE ( 'NONE', #23405, #14849, #9758, .T. ) ;
#7929=DIRECTION ( 'NONE',  ( 1.000000000000000000, -0.000000000000000000, -0.000000000000000000 ) ) ;
#7962=ORIENTED_EDGE ( 'NONE', *, *, #1054, .T. ) ;
#7964=CARTESIAN_POINT ( 'NONE',  ( 95.59906517536109050, 155.0000000000000000, -31.00000000000000000 ) ) ;
#8003=ORIENTED_EDGE ( 'NONE', *, *, #12373, .T. ) ;
#8004=CIRCLE ( 'NONE', #12346, 12.99999999999998401 ) ;
#8015=CIRCLE ( 'NONE', #25955, 32.10452846326769816 ) ;
#8043=AXIS2_PLACEMENT_3D ( 'NONE', #5274, #31021, #13114 ) ;
#8054=CIRCLE ( 'NONE', #1493, 32.00000000000000000 ) ;
#8061=DIRECTION ( 'NONE',  ( 0.000000000000000000, 0.000000000000000000, -1.000000000000000000 ) ) ;
#8066=LINE ( 'NONE', #20675, #13150 ) ;
#8072=CIRCLE ( 'NONE', #18920, 32.10452846326769816 ) ;
#8079=DIRECTION ( 'NONE',  ( 1.000000000000000000, -0.000000000000000000, -0.000000000000000000 ) ) ;
#8093=AXIS2_PLACEMENT_3D ( 'NONE', #4131, #16743, #24420 ) ;
#8106=CARTESIAN_POINT ( 'NONE',  ( 92.60756280994512224, 155.0000000000000000, -12.10452846326762177 ) ) ;
#8132=VERTEX_POINT ( 'NONE', #22010 ) ;
#8141=ADVANCED_FACE ( 'NONE', ( #25238 ), #1605, .F. ) ;
#8147=EDGE_CURVE ( 'NONE', #33389, #21429, #1225, .T. ) ;
#8202=ORIENTED_EDGE ( 'NONE', *, *, #10868, .F. ) ;
#8207=EDGE_LOOP ( 'NONE', ( #18147, #28369, #4988, #23570 ) ) ;
#8209=ORIENTED_EDGE ( 'NONE', *, *, #7715, .T. ) ;
#8218=DIRECTION ( 'NONE',  ( -1.000000000000000000, 0.000000000000000000, 0.000000000000000000 ) ) ;
#8228=DIRECTION ( 'NONE',  ( 0.000000000000000000, 0.000000000000000000, -1.000000000000000000 ) ) ;
#8234=DIRECTION ( 'NONE',  ( 1.000000000000000000, -0.000000000000000000, -0.000000000000000000 ) ) ;
#8236=CARTESIAN_POINT ( 'NONE',  ( 89.50000000000002842, 155.0000000000000000, 0.000000000000000000 ) ) ;
#8252=VERTEX_POINT ( 'NONE', #30014 ) ;
#8275=EDGE_CURVE ( 'NONE', #16362, #546, #17569, .T. ) ;
#8280=FACE_OUTER_BOUND ( 'NONE', #3869, .T. ) ;
#8294=EDGE_CURVE ( 'NONE', #8132, #2210, #19551, .T. ) ;
#8295=AXIS2_PLACEMENT_3D ( 'NONE', #9450, #22388, #1612 ) ;
#8299=DIRECTION ( 'NONE',  ( 1.000000000000000000, -0.000000000000000000, -0.000000000000000000 ) ) ;
#8305=DIRECTION ( 'NONE',  ( 0.000000000000000000, 0.000000000000000000, 1.000000000000000000 ) ) ;
#8334=EDGE_CURVE ( 'NONE', #16034, #8252, #23367, .T. ) ;
#8409=DIRECTION ( 'NONE',  ( -1.000000000000000000, 0.000000000000000000, 0.000000000000000000 ) ) ;
#8426=DIRECTION ( 'NONE',  ( 1.000000000000000000, -0.000000000000000000, -0.000000000000000000 ) ) ;
#8436=DIRECTION ( 'NONE',  ( 0.000000000000000000, 0.000000000000000000, -1.000000000000000000 ) ) ;
#8464=DIRECTION ( 'NONE',  ( 1.000000000000000000, -0.000000000000000000, -0.000000000000000000 ) ) ;
#8509=EDGE_CURVE ( 'NONE', #26453, #31583, #15852, .T. ) ;
#8514=AXIS2_PLACEMENT_3D ( 'NONE', #15063, #14558, #4340 ) ;
#8522=DIRECTION ( 'NONE',  ( 1.000000000000000000, -0.000000000000000000, -0.000000000000000000 ) ) ;
#8529=EDGE_LOOP ( 'NONE', ( #10613, #15556, #22875, #2463 ) ) ;
#8546=EDGE_CURVE ( 'NONE', #12687, #31608, #16285, .T. ) ;
#8563=AXIS2_PLACEMENT_3D ( 'NONE', #4613, #6655, #4433 ) ;
#8575=ORIENTED_EDGE ( 'NONE', *, *, #23263, .F. ) ;
#8652=ORIENTED_EDGE ( 'NONE', *, *, #1394, .T. ) ;
#8697=ORIENTED_EDGE ( 'NONE', *, *, #27673, .T. ) ;
#8707=ORIENTED_EDGE ( 'NONE', *, *, #21173, .T. ) ;
#8711=DIRECTION ( 'NONE',  ( 0.000000000000000000, 0.000000000000000000, -1.000000000000000000 ) ) ;
#8720=CARTESIAN_POINT ( 'NONE',  ( 97.30927364589244632, 155.0000000000000000, 31.00000000000000000 ) ) ;
#8778=FACE_OUTER_BOUND ( 'NONE', #29996, .T. ) ;
#8784=CONICAL_SURFACE ( 'NONE', #11516, 32.00000000000002842, 1.466076571675244411 ) ;
#8788=AXIS2_PLACEMENT_3D ( 'NONE', #22196, #25260, #14864 ) ;
#8826=DIRECTION ( 'NONE',  ( 0.000000000000000000, 0.000000000000000000, 1.000000000000000000 ) ) ;
#8840=AXIS2_PLACEMENT_3D ( 'NONE', #18667, #5710, #20553 ) ;
#8858=DIRECTION ( 'NONE',  ( 1.000000000000000000, -0.000000000000000000, -0.000000000000000000 ) ) ;
#8872=CARTESIAN_POINT ( 'NONE',  ( 0.000000000000000000, 0.000000000000000000, 0.000000000000000000 ) ) ;
#8880=AXIS2_PLACEMENT_3D ( 'NONE', #12418, #10384, #11928 ) ;
#8913=ORIENTED_EDGE ( 'NONE', *, *, #23263, .T. ) ;
#8920=DIRECTION ( 'NONE',  ( 0.000000000000000000, 0.000000000000000000, -1.000000000000000000 ) ) ;
#8932=LINE ( 'NONE', #10988, #21154 ) ;
#8943=CARTESIAN_POINT ( 'NONE',  ( 103.4083388212532810, 155.0000000000000000, -32.00000000000002842 ) ) ;
#8971=CARTESIAN_POINT ( 'NONE',  ( 107.9108275708642850, 155.0000000000000000, -13.00000000000001066 ) ) ;
#8995=CARTESIAN_POINT ( 'NONE',  ( 89.50000000000002842, 155.0000000000000000, -32.00000000000002842 ) ) ;
#9050=CARTESIAN_POINT ( 'NONE',  ( 98.19869130599479945, 155.0000000000000000, 0.000000000000000000 ) ) ;
#9052=FACE_OUTER_BOUND ( 'NONE', #21969, .T. ) ;
#9062=EDGE_CURVE ( 'NONE', #19467, #29217, #28824, .T. ) ;
#9093=VECTOR ( 'NONE', #22792, 1000.000000000000114 ) ;
#9110=VERTEX_POINT ( 'NONE', #3316 ) ;
#9120=ORIENTED_EDGE ( 'NONE', *, *, #26148, .F. ) ;
#9123=ADVANCED_FACE ( 'NONE', ( #3650 ), #1482, .F. ) ;
#9134=CARTESIAN_POINT ( 'NONE',  ( 97.20416941062678973, 155.0000000000000000, 32.00000000000000000 ) ) ;
#9153=ORIENTED_EDGE ( 'NONE', *, *, #12373, .F. ) ;
#9156=EDGE_LOOP ( 'NONE', ( #8202, #28007, #19707, #25965 ) ) ;
#9158=EDGE_CURVE ( 'NONE', #546, #10473, #8015, .T. ) ;
#9174=CARTESIAN_POINT ( 'NONE',  ( 92.60208470531341618, 155.0000000000000000, 0.000000000000000000 ) ) ;
#9257=DIRECTION ( 'NONE',  ( 0.000000000000000000, 0.000000000000000000, -1.000000000000000000 ) ) ;
#9268=DIRECTION ( 'NONE',  ( -0.9945218953682714025, 1.280104479605462180E-17, -0.1045284632676720116 ) ) ;
#9271=CARTESIAN_POINT ( 'NONE',  ( 108.0159016311981759, 155.0000000000000000, 0.000000000000000000 ) ) ;
#9330=ORIENTED_EDGE ( 'NONE', *, *, #8509, .T. ) ;
#9332=( NAMED_UNIT ( * ) PLANE_ANGLE_UNIT ( ) SI_UNIT ( $, .RADIAN. ) );
#9355=ORIENTED_EDGE ( 'NONE', *, *, #15223, .T. ) ;
#9371=CARTESIAN_POINT ( 'NONE',  ( 92.60208470531341618, 155.0000000000000000, 0.000000000000000000 ) ) ;
#9399=EDGE_LOOP ( 'NONE', ( #9153, #22321, #6718, #15357 ) ) ;
#9418=ORIENTED_EDGE ( 'NONE', *, *, #26864, .T. ) ;
#9422=CONICAL_SURFACE ( 'NONE', #5071, 32.10452846326769816, 1.466076571675243523 ) ;
#9437=AXIS2_PLACEMENT_3D ( 'NONE', #7797, #290, #18016 ) ;
#9450=CARTESIAN_POINT ( 'NONE',  ( 89.50000000000002842, 155.0000000000000000, 0.000000000000000000 ) ) ;
#9463=FACE_OUTER_BOUND ( 'NONE', #27830, .T. ) ;
#9493=ADVANCED_FACE ( 'NONE', ( #32376 ), #6144, .T. ) ;
#9494=ORIENTED_EDGE ( 'NONE', *, *, #22652, .T. ) ;
#9502=DIRECTION ( 'NONE',  ( -1.000000000000000000, 0.000000000000000000, 0.000000000000000000 ) ) ;
#9520=DIRECTION ( 'NONE',  ( 0.000000000000000000, 0.000000000000000000, -1.000000000000000000 ) ) ;
#9530=DIRECTION ( 'NONE',  ( 0.000000000000000000, 0.000000000000000000, -1.000000000000000000 ) ) ;
#9536=ORIENTED_EDGE ( 'NONE', *, *, #29925, .F. ) ;
#9555=FACE_OUTER_BOUND ( 'NONE', #24823, .T. ) ;
#9564=ORIENTED_EDGE ( 'NONE', *, *, #31812, .T. ) ;
#9595=ADVANCED_BREP_SHAPE_REPRESENTATION ( '', ( #11828, #2404 ), #30714 ) ;
#9597=LINE ( 'NONE', #20160, #24890 ) ;
#9598=LINE ( 'NONE', #11987, #32969 ) ;
#9617=DIRECTION ( 'NONE',  ( 1.000000000000000000, -0.000000000000000000, -0.000000000000000000 ) ) ;
#9642=CARTESIAN_POINT ( 'NONE',  ( 92.59660660068168170, 155.0000000000000000, 0.000000000000000000 ) ) ;
#9678=EDGE_CURVE ( 'NONE', #18054, #26344, #11940, .T. ) ;
#9701=DIRECTION ( 'NONE',  ( 1.000000000000000000, -0.000000000000000000, -0.000000000000000000 ) ) ;
#9745=DIRECTION ( 'NONE',  ( -0.1045284632676468234, 0.000000000000000000, 0.9945218953682740670 ) ) ;
#9752=EDGE_CURVE ( 'NONE', #5220, #29148, #24306, .T. ) ;
#9758=CIRCLE ( 'NONE', #31524, 13.00000000000001066 ) ;
#9788=ORIENTED_EDGE ( 'NONE', *, *, #14980, .T. ) ;
#9797=DIRECTION ( 'NONE',  ( -0.9945218953682777308, 1.280104479604737106E-17, -0.1045284632676128089 ) ) ;
#9839=ORIENTED_EDGE ( 'NONE', *, *, #6430, .F. ) ;
#9852=CARTESIAN_POINT ( 'NONE',  ( 91.60208470531341618, 155.0000000000000000, -12.00000000000001066 ) ) ;
#9882=DIRECTION ( 'NONE',  ( 1.000000000000000000, -0.000000000000000000, -0.000000000000000000 ) ) ;
#9926=VERTEX_POINT ( 'NONE', #10730 ) ;
#9967=ADVANCED_FACE ( 'NONE', ( #28791 ), #3665, .F. ) ;
#10024=CYLINDRICAL_SURFACE ( 'NONE', #9437, 32.00000000000002842 ) ;
#10027=EDGE_CURVE ( 'NONE', #17374, #2210, #10572, .T. ) ;
#10029=ORIENTED_EDGE ( 'NONE', *, *, #10643, .T. ) ;
#10059=ORIENTED_EDGE ( 'NONE', *, *, #4099, .F. ) ;
#10090=DIRECTION ( 'NONE',  ( 0.000000000000000000, 0.000000000000000000, 1.000000000000000000 ) ) ;
#10092=DIRECTION ( 'NONE',  ( 1.000000000000000000, -0.000000000000000000, -0.000000000000000000 ) ) ;
#10105=ORIENTED_EDGE ( 'NONE', *, *, #8509, .F. ) ;
#10117=DIRECTION ( 'NONE',  ( 0.000000000000000000, 0.000000000000000000, -1.000000000000000000 ) ) ;
#10139=LINE ( 'NONE', #30924, #3415 ) ;
#10145=EDGE_LOOP ( 'NONE', ( #13224, #13843, #20442, #28499 ) ) ;
#10171=FACE_OUTER_BOUND ( 'NONE', #30702, .T. ) ;
#10177=ORIENTED_EDGE ( 'NONE', *, *, #24157, .T. ) ;
#10183=EDGE_LOOP ( 'NONE', ( #23247, #11254, #20346, #5861 ) ) ;
#10213=AXIS2_PLACEMENT_3D ( 'NONE', #4377, #17663, #1993 ) ;
#10273=CIRCLE ( 'NONE', #29851, 32.00000000000000000 ) ;
#10280=CARTESIAN_POINT ( 'NONE',  ( 89.50000000000002842, 155.0000000000000000, 0.000000000000000000 ) ) ;
#10316=EDGE_LOOP ( 'NONE', ( #26793, #21061, #3744, #244 ) ) ;
#10322=ORIENTED_EDGE ( 'NONE', *, *, #25212, .T. ) ;
#10338=CARTESIAN_POINT ( 'NONE',  ( 100.3117322205716420, 155.0000000000000000, 0.000000000000000000 ) ) ;
#10343=DIRECTION ( 'NONE',  ( 0.000000000000000000, 0.000000000000000000, 1.000000000000000000 ) ) ;
#10367=LINE ( 'NONE', #22960, #33620 ) ;
#10384=DIRECTION ( 'NONE',  ( 1.000000000000000000, -0.000000000000000000, -0.000000000000000000 ) ) ;
#10392=DIRECTION ( 'NONE',  ( 0.000000000000000000, 0.000000000000000000, -1.000000000000000000 ) ) ;
#10412=ADVANCED_FACE ( 'NONE', ( #30120 ), #17167, .F. ) ;
#10433=DIRECTION ( 'NONE',  ( 1.000000000000000000, -0.000000000000000000, -0.000000000000000000 ) ) ;
#10436=ORIENTED_EDGE ( 'NONE', *, *, #767, .F. ) ;
#10455=CARTESIAN_POINT ( 'NONE',  ( 93.60208470531338776, 155.0000000000000000, 0.000000000000000000 ) ) ;
#10464=ADVANCED_FACE ( 'NONE', ( #32837 ), #11290, .F. ) ;
#10472=DIRECTION ( 'NONE',  ( 0.000000000000000000, 0.000000000000000000, -1.000000000000000000 ) ) ;
#10473=VERTEX_POINT ( 'NONE', #33004 ) ;
#10487=EDGE_LOOP ( 'NONE', ( #14939, #1996, #15165, #9839 ) ) ;
#10517=ORIENTED_EDGE ( 'NONE', *, *, #27513, .F. ) ;
#10560=ORIENTED_EDGE ( 'NONE', *, *, #27240, .T. ) ;
#10572=LINE ( 'NONE', #2397, #5850 ) ;
#10587=DIRECTION ( 'NONE',  ( 0.000000000000000000, 0.000000000000000000, 1.000000000000000000 ) ) ;
#10597=ORIENTED_EDGE ( 'NONE', *, *, #12033, .F. ) ;
#10613=ORIENTED_EDGE ( 'NONE', *, *, #33487, .T. ) ;
#10631=ORIENTED_EDGE ( 'NONE', *, *, #23137, .F. ) ;
#10635=DIRECTION ( 'NONE',  ( 1.000000000000000000, -0.000000000000000000, -0.000000000000000000 ) ) ;
#10643=EDGE_CURVE ( 'NONE', #16362, #32773, #10367, .T. ) ;
#10677=ORIENTED_EDGE ( 'NONE', *, *, #30798, .F. ) ;
#10697=CARTESIAN_POINT ( 'NONE',  ( 110.1179863365115636, 155.0000000000000000, 32.10452846326764131 ) ) ;
#10729=ORIENTED_EDGE ( 'NONE', *, *, #15768, .F. ) ;
#10730=CARTESIAN_POINT ( 'NONE',  ( 105.9028607166213192, 155.0000000000000000, 32.10452846326769816 ) ) ;
#10740=VECTOR ( 'NONE', #2850, 1000.000000000000000 ) ;
#10755=ORIENTED_EDGE ( 'NONE', *, *, #18143, .T. ) ;
#10777=CYLINDRICAL_SURFACE ( 'NONE', #27324, 32.00000000000001421 ) ;
#10805=FACE_OUTER_BOUND ( 'NONE', #984, .T. ) ;
#10816=FACE_OUTER_BOUND ( 'NONE', #8207, .T. ) ;
#10822=CONICAL_SURFACE ( 'NONE', #6458, 32.10452846326769816, 1.466076571675243523 ) ;
#10835=CARTESIAN_POINT ( 'NONE',  ( 103.4083388212532810, 155.0000000000000000, 0.000000000000000000 ) ) ;
#10841=AXIS2_PLACEMENT_3D ( 'NONE', #13987, #32048, #8711 ) ;
#10861=LINE ( 'NONE', #954, #12408 ) ;
#10868=EDGE_CURVE ( 'NONE', #82, #23658, #5565, .T. ) ;
#10869=DIRECTION ( 'NONE',  ( -0.1045284632676468234, 1.217938055844715641E-16, -0.9945218953682740670 ) ) ;
#10893=CARTESIAN_POINT ( 'NONE',  ( 92.60208470531341618, 155.0000000000000000, 12.10452846326763598 ) ) ;
#10948=CARTESIAN_POINT ( 'NONE',  ( 99.30625411593993590, 155.0000000000000000, -12.00000000000001066 ) ) ;
#10988=CARTESIAN_POINT ( 'NONE',  ( 111.1125082318798007, 155.0000000000000000, -32.00000000000002842 ) ) ;
#10996=CARTESIAN_POINT ( 'NONE',  ( 103.3032345859876102, 155.0000000000000000, 0.000000000000000000 ) ) ;
#11017=CONICAL_SURFACE ( 'NONE', #22980, 32.00000000000002842, 1.466076571675243523 ) ;
#11053=EDGE_CURVE ( 'NONE', #210, #17299, #15943, .T. ) ;
#11060=EDGE_CURVE ( 'NONE', #14849, #23405, #21919, .T. ) ;
#11078=CARTESIAN_POINT ( 'NONE',  ( 110.1179863365115636, 155.0000000000000000, 0.000000000000000000 ) ) ;
#11111=AXIS2_PLACEMENT_3D ( 'NONE', #21525, #14027, #8920 ) ;
#11138=CARTESIAN_POINT ( 'NONE',  ( 95.70416941062676131, 155.0000000000000000, -32.00000000000005684 ) ) ;
#11140=VERTEX_POINT ( 'NONE', #27484 ) ;
#11148=DIRECTION ( 'NONE',  ( 0.000000000000000000, 0.000000000000000000, -1.000000000000000000 ) ) ;
#11222=CARTESIAN_POINT ( 'NONE',  ( 100.3117322205716420, 155.0000000000000000, 12.10452846326767506 ) ) ;
#11246=ORIENTED_EDGE ( 'NONE', *, *, #11060, .T. ) ;
#11254=ORIENTED_EDGE ( 'NONE', *, *, #622, .F. ) ;
#11267=ORIENTED_EDGE ( 'NONE', *, *, #29550, .T. ) ;
#11290=CONICAL_SURFACE ( 'NONE', #31968, 31.00000000000000000, 1.466076571675243967 ) ;
#11318=DIRECTION ( 'NONE',  ( 0.000000000000000000, 0.000000000000000000, -1.000000000000000000 ) ) ;
#11341=CARTESIAN_POINT ( 'NONE',  ( 101.3062541159399075, 155.0000000000000000, 0.000000000000000000 ) ) ;
#11342=ORIENTED_EDGE ( 'NONE', *, *, #31819, .T. ) ;
#11378=ADVANCED_FACE ( 'NONE', ( #12828 ), #33368, .F. ) ;
#11388=CARTESIAN_POINT ( 'NONE',  ( 91.60208470531341618, 155.0000000000000000, 0.000000000000000000 ) ) ;
#11419=ORIENTED_EDGE ( 'NONE', *, *, #32456, .F. ) ;
#11430=ORIENTED_EDGE ( 'NONE', *, *, #29550, .F. ) ;
#11455=CARTESIAN_POINT ( 'NONE',  ( 107.0104235265664556, 155.0000000000000000, 11.99999999999998224 ) ) ;
#11459=DIRECTION ( 'NONE',  ( 1.000000000000000000, -0.000000000000000000, -0.000000000000000000 ) ) ;
#11467=AXIS2_PLACEMENT_3D ( 'NONE', #19947, #15006, #30346 ) ;
#11516=AXIS2_PLACEMENT_3D ( 'NONE', #12831, #24220, #29341 ) ;
#11541=EDGE_LOOP ( 'NONE', ( #11419, #31297, #3660, #29620 ) ) ;
#11551=LINE ( 'NONE', #8995, #17786 ) ;
#11559=LINE ( 'NONE', #29283, #19078 ) ;
#11569=CARTESIAN_POINT ( 'NONE',  ( 110.1179863365115636, 155.0000000000000000, -32.10452846326764131 ) ) ;
#11574=CARTESIAN_POINT ( 'NONE',  ( 97.20416941062678973, 155.0000000000000000, 0.000000000000000000 ) ) ;
#11582=DIRECTION ( 'NONE',  ( 0.000000000000000000, 0.000000000000000000, -1.000000000000000000 ) ) ;
#11612=LINE ( 'NONE', #18779, #30121 ) ;
#11726=CARTESIAN_POINT ( 'NONE',  ( 110.1179863365115636, 155.0000000000000000, 0.000000000000000000 ) ) ;
#11737=LINE ( 'NONE', #12073, #456 ) ;
#11749=CARTESIAN_POINT ( 'NONE',  ( 94.70964751525852421, 155.0000000000000000, 0.000000000000000000 ) ) ;
#11783=DIRECTION ( 'NONE',  ( 0.000000000000000000, 0.000000000000000000, -1.000000000000000000 ) ) ;
#11804=DIRECTION ( 'NONE',  ( -1.000000000000000000, 0.000000000000000000, 0.000000000000000000 ) ) ;
#11828=MANIFOLD_SOLID_BREP ( 'Revolve1', #6889 ) ;
#11833=VECTOR ( 'NONE', #8426, 1000.000000000000000 ) ;
#11857=DIRECTION ( 'NONE',  ( 1.000000000000000000, -0.000000000000000000, -0.000000000000000000 ) ) ;
#11887=EDGE_LOOP ( 'NONE', ( #10436, #22916, #14391, #23705 ) ) ;
#11893=CARTESIAN_POINT ( 'NONE',  ( 103.3032345859876102, 155.0000000000000000, 31.00000000000000000 ) ) ;
#11906=CIRCLE ( 'NONE', #27153, 32.00000000000002842 ) ;
#11912=DIRECTION ( 'NONE',  ( 0.000000000000000000, 0.000000000000000000, 1.000000000000000000 ) ) ;
#11928=DIRECTION ( 'NONE',  ( 0.000000000000000000, 0.000000000000000000, -1.000000000000000000 ) ) ;
#11940=LINE ( 'NONE', #4093, #29230 ) ;
#11941=DIRECTION ( 'NONE',  ( 0.000000000000000000, 0.000000000000000000, 1.000000000000000000 ) ) ;
#11987=CARTESIAN_POINT ( 'NONE',  ( 99.30625411593993590, 155.0000000000000000, 12.00000000000001066 ) ) ;
#12008=CYLINDRICAL_SURFACE ( 'NONE', #12948, 12.10452846326766441 ) ;
#12033=EDGE_CURVE ( 'NONE', #9926, #21869, #16523, .T. ) ;
#12073=CARTESIAN_POINT ( 'NONE',  ( 97.30927364589244632, 155.0000000000000000, 31.00000000000000000 ) ) ;
#12089=ORIENTED_EDGE ( 'NONE', *, *, #31845, .T. ) ;
#12111=SURFACE_STYLE_USAGE ( .BOTH. , #14664 ) ;
#12119=LINE ( 'NONE', #4280, #3146 ) ;
#12137=DIRECTION ( 'NONE',  ( 1.000000000000000000, -0.000000000000000000, -0.000000000000000000 ) ) ;
#12194=COLOUR_RGB ( '', 0.09019608, 0.27058824, 0.51372549) ;
#12210=CARTESIAN_POINT ( 'NONE',  ( 92.60208470531341618, 155.0000000000000000, 0.000000000000000000 ) ) ;
#12242=DIRECTION ( 'NONE',  ( 0.9945218953682689600, 1.280104479605745523E-17, 0.1045284632676951458 ) ) ;
#12256=FACE_OUTER_BOUND ( 'NONE', #28695, .T. ) ;
#12257=ORIENTED_EDGE ( 'NONE', *, *, #25979, .F. ) ;
#12258=ORIENTED_EDGE ( 'NONE', *, *, #12448, .F. ) ;
#12346=AXIS2_PLACEMENT_3D ( 'NONE', #748, #7929, #5849 ) ;
#12373=EDGE_CURVE ( 'NONE', #20431, #12687, #11612, .T. ) ;
#12390=ORIENTED_EDGE ( 'NONE', *, *, #21173, .F. ) ;
#12392=CONICAL_SURFACE ( 'NONE', #33086, 32.10452846326766974, 1.466076571675243523 ) ;
#12408=VECTOR ( 'NONE', #21401, 1000.000000000000114 ) ;
#12415=EDGE_CURVE ( 'NONE', #21262, #29530, #228, .T. ) ;
#12417=CIRCLE ( 'NONE', #1518, 32.00000000000000000 ) ;
#12418=CARTESIAN_POINT ( 'NONE',  ( 111.1125082318798007, 155.0000000000000000, 0.000000000000000000 ) ) ;
#12428=LINE ( 'NONE', #25370, #2030 ) ;
#12437=ORIENTED_EDGE ( 'NONE', *, *, #2730, .T. ) ;
#12448=EDGE_CURVE ( 'NONE', #21804, #889, #555, .T. ) ;
#12456=CONICAL_SURFACE ( 'NONE', #18995, 32.10452846326769816, 1.466076571675243079 ) ;
#12481=VECTOR ( 'NONE', #7698, 1000.000000000000000 ) ;
#12535=CARTESIAN_POINT ( 'NONE',  ( 92.50248874961125978, 155.0000000000000000, 0.000000000000000000 ) ) ;
#12551=CARTESIAN_POINT ( 'NONE',  ( 97.30927364589244632, 155.0000000000000000, 0.000000000000000000 ) ) ;
#12608=CARTESIAN_POINT ( 'NONE',  ( 103.3032345859876102, 155.0000000000000000, 0.000000000000000000 ) ) ;
#12624=FACE_OUTER_BOUND ( 'NONE', #84, .T. ) ;
#12654=CARTESIAN_POINT ( 'NONE',  ( 100.2066581602377653, 155.0000000000000000, 0.000000000000000000 ) ) ;
#12661=DIRECTION ( 'NONE',  ( 0.000000000000000000, 0.000000000000000000, 1.000000000000000000 ) ) ;
#12668=VECTOR ( 'NONE', #10635, 1000.000000000000000 ) ;
#12683=LINE ( 'NONE', #33470, #32792 ) ;
#12687=VERTEX_POINT ( 'NONE', #5287 ) ;
#12697=FACE_OUTER_BOUND ( 'NONE', #10183, .T. ) ;
#12726=CARTESIAN_POINT ( 'NONE',  ( 92.60208470531341618, 155.0000000000000000, 0.000000000000000000 ) ) ;
#12754=DIRECTION ( 'NONE',  ( 1.000000000000000000, -0.000000000000000000, -0.000000000000000000 ) ) ;
#12769=CYLINDRICAL_SURFACE ( 'NONE', #23235, 12.10452846326765020 ) ;
#12777=ORIENTED_EDGE ( 'NONE', *, *, #13635, .F. ) ;
#12788=( NAMED_UNIT ( * ) PLANE_ANGLE_UNIT ( ) SI_UNIT ( $, .RADIAN. ) );
#12811=ORIENTED_EDGE ( 'NONE', *, *, #14769, .F. ) ;
#12828=FACE_OUTER_BOUND ( 'NONE', #27882, .T. ) ;
#12831=CARTESIAN_POINT ( 'NONE',  ( 111.1125082318798007, 155.0000000000000000, 0.000000000000000000 ) ) ;
#12842=CARTESIAN_POINT ( 'NONE',  ( 92.60208470531341618, 155.0000000000000000, -12.10452846326766441 ) ) ;
#12878=DIRECTION ( 'NONE',  ( -1.000000000000000000, 0.000000000000000000, 0.000000000000000000 ) ) ;
#12889=ORIENTED_EDGE ( 'NONE', *, *, #33460, .F. ) ;
#12897=VECTOR ( 'NONE', #26052, 1000.000000000000000 ) ;
#12907=DIRECTION ( 'NONE',  ( 0.000000000000000000, 0.000000000000000000, -1.000000000000000000 ) ) ;
#12909=EDGE_CURVE ( 'NONE', #14059, #22749, #18193, .T. ) ;
#12933=CONICAL_SURFACE ( 'NONE', #7497, 32.10452846326769816, 1.466076571675243523 ) ;
#12948=AXIS2_PLACEMENT_3D ( 'NONE', #32784, #24625, #22394 ) ;
#12993=ORIENTED_EDGE ( 'NONE', *, *, #2095, .F. ) ;
#13114=DIRECTION ( 'NONE',  ( 0.000000000000000000, 0.000000000000000000, 1.000000000000000000 ) ) ;
#13139=ADVANCED_FACE ( 'NONE', ( #5417 ), #14394, .F. ) ;
#13150=VECTOR ( 'NONE', #29002, 1000.000000000000114 ) ;
#13224=ORIENTED_EDGE ( 'NONE', *, *, #9062, .F. ) ;
#13227=CONICAL_SURFACE ( 'NONE', #25729, 12.00000000000001066, 0.1047197551196188681 ) ;
#13247=VECTOR ( 'NONE', #31720, 1000.000000000000227 ) ;
#13294=ADVANCED_FACE ( 'NONE', ( #25693 ), #5246, .T. ) ;
#13337=ORIENTED_EDGE ( 'NONE', *, *, #23977, .F. ) ;
#13374=ORIENTED_EDGE ( 'NONE', *, *, #14915, .F. ) ;
#13424=CONICAL_SURFACE ( 'NONE', #32458, 32.10452846326766974, 1.466076571675243301 ) ;
#13429=DIRECTION ( 'NONE',  ( 0.000000000000000000, 0.000000000000000000, -1.000000000000000000 ) ) ;
#13459=ADVANCED_FACE ( 'NONE', ( #31801 ), #18751, .T. ) ;
#13460=DIRECTION ( 'NONE',  ( 1.000000000000000000, -0.000000000000000000, -0.000000000000000000 ) ) ;
#13493=CARTESIAN_POINT ( 'NONE',  ( 105.9028607166213192, 155.0000000000000000, -32.10452846326769816 ) ) ;
#13506=AXIS2_PLACEMENT_3D ( 'NONE', #9642, #19536, #19361 ) ;
#13554=EDGE_CURVE ( 'NONE', #26453, #14059, #17139, .T. ) ;
#13592=CARTESIAN_POINT ( 'NONE',  ( 91.60208470531341618, 155.0000000000000000, -12.00000000000001066 ) ) ;
#13608=CARTESIAN_POINT ( 'NONE',  ( 105.9028607166213192, 155.0000000000000000, 0.000000000000000000 ) ) ;
#13635=EDGE_CURVE ( 'NONE', #21429, #4805, #31657, .T. ) ;
#13668=CIRCLE ( 'NONE', #16951, 32.10452846326769816 ) ;
#13693=VECTOR ( 'NONE', #24473, 1000.000000000000114 ) ;
#13698=EDGE_CURVE ( 'NONE', #2210, #20526, #16964, .T. ) ;
#13701=ORIENTED_EDGE ( 'NONE', *, *, #20406, .F. ) ;
#13716=ORIENTED_EDGE ( 'NONE', *, *, #14920, .F. ) ;
#13736=DIRECTION ( 'NONE',  ( -1.000000000000000000, 0.000000000000000000, 0.000000000000000000 ) ) ;
#13739=DIRECTION ( 'NONE',  ( 0.000000000000000000, 0.000000000000000000, -1.000000000000000000 ) ) ;
#13774=DIRECTION ( 'NONE',  ( 1.000000000000000000, -0.000000000000000000, -0.000000000000000000 ) ) ;
#13786=DIRECTION ( 'NONE',  ( 0.000000000000000000, 0.000000000000000000, -1.000000000000000000 ) ) ;
#13793=CIRCLE ( 'NONE', #5099, 13.00000000000001066 ) ;
#13802=LINE ( 'NONE', #16028, #32995 ) ;
#13838=DIRECTION ( 'NONE',  ( 0.000000000000000000, 0.000000000000000000, -1.000000000000000000 ) ) ;
#13843=ORIENTED_EDGE ( 'NONE', *, *, #4058, .T. ) ;
#13855=EDGE_CURVE ( 'NONE', #15528, #4327, #6081, .T. ) ;
#13896=DIRECTION ( 'NONE',  ( -1.000000000000000000, 0.000000000000000000, 0.000000000000000000 ) ) ;
#13898=ADVANCED_FACE ( 'NONE', ( #25088 ), #7745, .T. ) ;
#13908=DIRECTION ( 'NONE',  ( 0.000000000000000000, 0.000000000000000000, -1.000000000000000000 ) ) ;
#13987=CARTESIAN_POINT ( 'NONE',  ( 92.60756280994512224, 155.0000000000000000, 0.000000000000000000 ) ) ;
#13995=DIRECTION ( 'NONE',  ( -0.1045284632676463932, 1.217938055844715641E-16, -0.9945218953682741780 ) ) ;
#14007=DIRECTION ( 'NONE',  ( 0.9945218953682747332, 0.000000000000000000, -0.1045284632676402453 ) ) ;
#14027=DIRECTION ( 'NONE',  ( 1.000000000000000000, -0.000000000000000000, -0.000000000000000000 ) ) ;
#14035=FACE_OUTER_BOUND ( 'NONE', #30793, .T. ) ;
#14039=EDGE_LOOP ( 'NONE', ( #29520, #14857, #15107, #20778 ) ) ;
#14059=VERTEX_POINT ( 'NONE', #4310 ) ;
#14073=AXIS2_PLACEMENT_3D ( 'NONE', #17984, #7423, #2483 ) ;
#14183=LINE ( 'NONE', #26456, #29013 ) ;
#14258=CARTESIAN_POINT ( 'NONE',  ( 101.3062541159399075, 155.0000000000000000, 12.00000000000001066 ) ) ;
#14289=CIRCLE ( 'NONE', #19179, 32.00000000000002842 ) ;
#14304=ORIENTED_EDGE ( 'NONE', *, *, #8147, .F. ) ;
#14308=ORIENTED_EDGE ( 'NONE', *, *, #8275, .F. ) ;
#14315=CIRCLE ( 'NONE', #7251, 12.00000000000001066 ) ;
#14358=ADVANCED_FACE ( 'NONE', ( #15874 ), #11017, .F. ) ;
#14361=ORIENTED_EDGE ( 'NONE', *, *, #28569, .F. ) ;
#14391=ORIENTED_EDGE ( 'NONE', *, *, #9678, .T. ) ;
#14394=CONICAL_SURFACE ( 'NONE', #31792, 11.99999999999998224, 0.1047197551197030924 ) ;
#14414=DIRECTION ( 'NONE',  ( 0.1045284632676459352, 0.000000000000000000, -0.9945218953682740670 ) ) ;
#14441=LINE ( 'NONE', #11893, #9093 ) ;
#14443=ORIENTED_EDGE ( 'NONE', *, *, #17799, .F. ) ;
#14456=CARTESIAN_POINT ( 'NONE',  ( 111.1125082318798007, 155.0000000000000000, 0.000000000000000000 ) ) ;
#14478=ADVANCED_FACE ( 'NONE', ( #23712 ), #10777, .T. ) ;
#14497=CARTESIAN_POINT ( 'NONE',  ( 101.3062541159399075, 155.0000000000000000, 0.000000000000000000 ) ) ;
#14500=VECTOR ( 'NONE', #2942, 1000.000000000000000 ) ;
#14511=DIRECTION ( 'NONE',  ( 0.000000000000000000, 0.000000000000000000, -1.000000000000000000 ) ) ;
#14513=ADVANCED_FACE ( 'NONE', ( #29155 ), #23516, .F. ) ;
#14539=DIRECTION ( 'NONE',  ( -1.000000000000000000, 0.000000000000000000, 0.000000000000000000 ) ) ;
#14558=DIRECTION ( 'NONE',  ( 1.000000000000000000, -0.000000000000000000, -0.000000000000000000 ) ) ;
#14588=EDGE_CURVE ( 'NONE', #26664, #17299, #24039, .T. ) ;
#14602=ORIENTED_EDGE ( 'NONE', *, *, #27889, .F. ) ;
#14604=EDGE_LOOP ( 'NONE', ( #26103, #10322, #9330, #12811 ) ) ;
#14607=ORIENTED_EDGE ( 'NONE', *, *, #17512, .T. ) ;
#14664=SURFACE_SIDE_STYLE ('',( #4271 ) ) ;
#14669=DIRECTION ( 'NONE',  ( 1.000000000000000000, -0.000000000000000000, -0.000000000000000000 ) ) ;
#14716=EDGE_CURVE ( 'NONE', #22749, #14059, #3925, .T. ) ;
#14731=VERTEX_POINT ( 'NONE', #16797 ) ;
#14766=ORIENTED_EDGE ( 'NONE', *, *, #26879, .F. ) ;
#14769=EDGE_CURVE ( 'NONE', #27125, #31583, #16979, .T. ) ;
#14774=ADVANCED_FACE ( 'NONE', ( #3346 ), #126, .T. ) ;
#14816=DIRECTION ( 'NONE',  ( 1.000000000000000000, -0.000000000000000000, -0.000000000000000000 ) ) ;
#14819=EDGE_LOOP ( 'NONE', ( #13716, #5264, #30491, #6563 ) ) ;
#14822=AXIS2_PLACEMENT_3D ( 'NONE', #29586, #8464, #23800 ) ;
#14849=VERTEX_POINT ( 'NONE', #631 ) ;
#14850=AXIS2_PLACEMENT_3D ( 'NONE', #12535, #31442, #28210 ) ;
#14857=ORIENTED_EDGE ( 'NONE', *, *, #15294, .F. ) ;
#14864=DIRECTION ( 'NONE',  ( 0.000000000000000000, 0.000000000000000000, 1.000000000000000000 ) ) ;
#14889=DIRECTION ( 'NONE',  ( 0.000000000000000000, 0.000000000000000000, -1.000000000000000000 ) ) ;
#14895=DIRECTION ( 'NONE',  ( 1.000000000000000000, -0.000000000000000000, -0.000000000000000000 ) ) ;
#14897=EDGE_LOOP ( 'NONE', ( #10059, #26063, #20439, #1622 ) ) ;
#14915=EDGE_CURVE ( 'NONE', #21869, #9926, #1204, .T. ) ;
#14920=EDGE_CURVE ( 'NONE', #14849, #3157, #27194, .T. ) ;
#14939=ORIENTED_EDGE ( 'NONE', *, *, #18522, .F. ) ;
#14967=CARTESIAN_POINT ( 'NONE',  ( 104.9083388212530537, 155.0000000000000000, 32.00000000000000000 ) ) ;
#14972=LINE ( 'NONE', #22812, #23046 ) ;
#14977=ORIENTED_EDGE ( 'NONE', *, *, #9158, .F. ) ;
#14980=EDGE_CURVE ( 'NONE', #29217, #6439, #17646, .T. ) ;
#14991=DIRECTION ( 'NONE',  ( 0.000000000000000000, 0.000000000000000000, -1.000000000000000000 ) ) ;
#15006=DIRECTION ( 'NONE',  ( -1.000000000000000000, 0.000000000000000000, 0.000000000000000000 ) ) ;
#15023=EDGE_LOOP ( 'NONE', ( #19499, #17582, #11267, #26931 ) ) ;
#15048=DIRECTION ( 'NONE',  ( 1.000000000000000000, -0.000000000000000000, -0.000000000000000000 ) ) ;
#15063=CARTESIAN_POINT ( 'NONE',  ( 110.1179863365115636, 155.0000000000000000, 0.000000000000000000 ) ) ;
#15072=ORIENTED_EDGE ( 'NONE', *, *, #23977, .T. ) ;
#15107=ORIENTED_EDGE ( 'NONE', *, *, #8334, .T. ) ;
#15111=CONICAL_SURFACE ( 'NONE', #15676, 12.00000000000001066, 0.1047197551196740739 ) ;
#15134=CARTESIAN_POINT ( 'NONE',  ( 109.0104235265664272, 155.0000000000000000, -11.99999999999998224 ) ) ;
#15139=DIRECTION ( 'NONE',  ( 0.9945218953682689600, 0.000000000000000000, -0.1045284632676951458 ) ) ;
#15161=DIRECTION ( 'NONE',  ( 1.000000000000000000, -0.000000000000000000, -0.000000000000000000 ) ) ;
#15165=ORIENTED_EDGE ( 'NONE', *, *, #19799, .T. ) ;
#15185=CIRCLE ( 'NONE', #22247, 31.00000000000000000 ) ;
#15223=EDGE_CURVE ( 'NONE', #17374, #11140, #30075, .T. ) ;
#15236=DIRECTION ( 'NONE',  ( 0.000000000000000000, 0.000000000000000000, -1.000000000000000000 ) ) ;
#15260=CARTESIAN_POINT ( 'NONE',  ( 97.30927364589244632, 155.0000000000000000, 0.000000000000000000 ) ) ;
#15294=EDGE_CURVE ( 'NONE', #16034, #14731, #15395, .T. ) ;
#15300=DIRECTION ( 'NONE',  ( 1.000000000000000000, -0.000000000000000000, -0.000000000000000000 ) ) ;
#15354=CARTESIAN_POINT ( 'NONE',  ( 103.4083388212532810, 155.0000000000000000, 32.00000000000002842 ) ) ;
#15357=ORIENTED_EDGE ( 'NONE', *, *, #8546, .F. ) ;
#15395=CIRCLE ( 'NONE', #14850, 13.00000000000001066 ) ;
#15398=CONICAL_SURFACE ( 'NONE', #701, 12.00000000000001066, 0.1047197551196740739 ) ;
#15411=ORIENTED_EDGE ( 'NONE', *, *, #1054, .F. ) ;
#15414=ORIENTED_EDGE ( 'NONE', *, *, #9678, .F. ) ;
#15438=EDGE_CURVE ( 'NONE', #23382, #17270, #31704, .T. ) ;
#15468=DIRECTION ( 'NONE',  ( 1.000000000000000000, -0.000000000000000000, -0.000000000000000000 ) ) ;
#15520=CARTESIAN_POINT ( 'NONE',  ( 97.20416941062678973, 155.0000000000000000, 0.000000000000000000 ) ) ;
#15528=VERTEX_POINT ( 'NONE', #4154 ) ;
#15556=ORIENTED_EDGE ( 'NONE', *, *, #18522, .T. ) ;
#15616=AXIS2_PLACEMENT_3D ( 'NONE', #9371, #14816, #14991 ) ;
#15621=EDGE_CURVE ( 'NONE', #4805, #23382, #2288, .T. ) ;
#15676=AXIS2_PLACEMENT_3D ( 'NONE', #14497, #22849, #1897 ) ;
#15726=VECTOR ( 'NONE', #18068, 1000.000000000000227 ) ;
#15768=EDGE_CURVE ( 'NONE', #26664, #28067, #3952, .T. ) ;
#15780=ORIENTED_EDGE ( 'NONE', *, *, #2735, .F. ) ;
#15802=DIRECTION ( 'NONE',  ( 0.000000000000000000, 0.000000000000000000, -1.000000000000000000 ) ) ;
#15813=ADVANCED_FACE ( 'NONE', ( #25451 ), #1787, .T. ) ;
#15820=AXIS2_PLACEMENT_3D ( 'NONE', #32001, #26893, #8826 ) ;
#15852=LINE ( 'NONE', #196, #26622 ) ;
#15855=ORIENTED_EDGE ( 'NONE', *, *, #7429, .T. ) ;
#15858=UNCERTAINTY_MEASURE_WITH_UNIT (LENGTH_MEASURE( 1.000000000000000082E-05 ), #32334, 'distance_accuracy_value', 'NONE');
#15874=FACE_OUTER_BOUND ( 'NONE', #11887, .T. ) ;
#15923=ORIENTED_EDGE ( 'NONE', *, *, #18090, .F. ) ;
#15933=CIRCLE ( 'NONE', #27894, 13.00000000000003908 ) ;
#15943=CIRCLE ( 'NONE', #29565, 32.10452846326766974 ) ;
#15958=VECTOR ( 'NONE', #23596, 1000.000000000000114 ) ;
#15969=MECHANICAL_DESIGN_GEOMETRIC_PRESENTATION_REPRESENTATION('',(#30672),#1285);
#16000=SURFACE_STYLE_USAGE ( .BOTH. , #5608 ) ;
#16015=ADVANCED_FACE ( 'NONE', ( #29179 ), #20874, .T. ) ;
#16025=EDGE_CURVE ( 'NONE', #25247, #26926, #18624, .T. ) ;
#16028=CARTESIAN_POINT ( 'NONE',  ( 92.60208470531341618, 155.0000000000000000, -13.00000000000002487 ) ) ;
#16034=VERTEX_POINT ( 'NONE', #19290 ) ;
#16053=ADVANCED_FACE ( 'NONE', ( #18790 ), #33398, .F. ) ;
#16063=DIRECTION ( 'NONE',  ( -1.000000000000000000, 0.000000000000000000, 0.000000000000000000 ) ) ;
#16069=ORIENTED_EDGE ( 'NONE', *, *, #17512, .F. ) ;
#16141=LINE ( 'NONE', #13592, #12897 ) ;
#16147=AXIS2_PLACEMENT_3D ( 'NONE', #28864, #5520, #11148 ) ;
#16165=PRODUCT_CONTEXT ( 'NONE', #2018, 'mechanical' ) ;
#16169=DIRECTION ( 'NONE',  ( 1.000000000000000000, -0.000000000000000000, -0.000000000000000000 ) ) ;
#16181=ORIENTED_EDGE ( 'NONE', *, *, #4058, .F. ) ;
#16205=FACE_OUTER_BOUND ( 'NONE', #32956, .T. ) ;
#16247=ORIENTED_EDGE ( 'NONE', *, *, #14920, .T. ) ;
#16249=EDGE_CURVE ( 'NONE', #23405, #20526, #27621, .T. ) ;
#16281=ORIENTED_EDGE ( 'NONE', *, *, #29925, .T. ) ;
#16285=CIRCLE ( 'NONE', #20662, 31.00000000000000000 ) ;
#16326=CARTESIAN_POINT ( 'NONE',  ( 111.1125082318798007, 155.0000000000000000, 0.000000000000000000 ) ) ;
#16332=SHAPE_DEFINITION_REPRESENTATION ( #27928, #17605 ) ;
#16350=CARTESIAN_POINT ( 'NONE',  ( 92.59660660068168170, 155.0000000000000000, -12.10452846326765020 ) ) ;
#16351=EDGE_LOOP ( 'NONE', ( #116, #8707, #1085, #31422 ) ) ;
#16362=VERTEX_POINT ( 'NONE', #17235 ) ;
#16364=DIRECTION ( 'NONE',  ( 0.000000000000000000, 0.000000000000000000, -1.000000000000000000 ) ) ;
#16378=DIRECTION ( 'NONE',  ( 0.000000000000000000, 0.000000000000000000, -1.000000000000000000 ) ) ;
#16437=DIRECTION ( 'NONE',  ( -1.000000000000000000, 0.000000000000000000, 0.000000000000000000 ) ) ;
#16444=FACE_OUTER_BOUND ( 'NONE', #28412, .T. ) ;
#16457=CARTESIAN_POINT ( 'NONE',  ( 105.9028607166213192, 155.0000000000000000, 0.000000000000000000 ) ) ;
#16523=CIRCLE ( 'NONE', #4004, 32.10452846326769816 ) ;
#16525=EDGE_LOOP ( 'NONE', ( #8575, #9418, #2092, #14977 ) ) ;
#16570=PRODUCT_DEFINITION_CONTEXT ( 'detailed design', #916, 'design' ) ;
#16585=ADVANCED_FACE ( 'NONE', ( #7367 ), #30130, .T. ) ;
#16601=CARTESIAN_POINT ( 'NONE',  ( 95.70416941062676131, 155.0000000000000000, 32.00000000000005684 ) ) ;
#16663=DIRECTION ( 'NONE',  ( 0.000000000000000000, 0.000000000000000000, -1.000000000000000000 ) ) ;
#16678=AXIS2_PLACEMENT_3D ( 'NONE', #22477, #6809, #32868 ) ;
#16698=AXIS2_PLACEMENT_3D ( 'NONE', #18330, #28724, #5381 ) ;
#16716=DIRECTION ( 'NONE',  ( 0.000000000000000000, 0.000000000000000000, -1.000000000000000000 ) ) ;
#16732=FACE_OUTER_BOUND ( 'NONE', #14604, .T. ) ;
#16743=DIRECTION ( 'NONE',  ( 1.000000000000000000, -0.000000000000000000, -0.000000000000000000 ) ) ;
#16775=CIRCLE ( 'NONE', #2103, 13.00000000000003908 ) ;
#16797=CARTESIAN_POINT ( 'NONE',  ( 92.50248874961125978, 155.0000000000000000, -13.00000000000001066 ) ) ;
#16799=DIRECTION ( 'NONE',  ( 0.9945218953682661844, 1.280104479606063378E-17, 0.1045284632677211112 ) ) ;
#16846=LINE ( 'NONE', #14967, #21120 ) ;
#16888=EDGE_CURVE ( 'NONE', #14731, #26926, #6293, .T. ) ;
#16890=EDGE_LOOP ( 'NONE', ( #23285, #25109, #27933, #17383 ) ) ;
#16916=FACE_OUTER_BOUND ( 'NONE', #931, .T. ) ;
#16938=DIRECTION ( 'NONE',  ( 0.000000000000000000, 0.000000000000000000, -1.000000000000000000 ) ) ;
#16941=ADVANCED_FACE ( 'NONE', ( #20212 ), #30268, .F. ) ;
#16951=AXIS2_PLACEMENT_3D ( 'NONE', #9050, #21663, #31884 ) ;
#16964=LINE ( 'NONE', #9134, #20789 ) ;
#16979=CIRCLE ( 'NONE', #25703, 12.10452846326762177 ) ;
#17007=AXIS2_PLACEMENT_3D ( 'NONE', #9271, #6549, #14889 ) ;
#17080=CIRCLE ( 'NONE', #11111, 13.00000000000001066 ) ;
#17085=ADVANCED_FACE ( 'NONE', ( #8280 ), #23113, .T. ) ;
#17104=CARTESIAN_POINT ( 'NONE',  ( 98.19869130599479945, 155.0000000000000000, 0.000000000000000000 ) ) ;
#17107=MECHANICAL_DESIGN_GEOMETRIC_PRESENTATION_REPRESENTATION('',(#32320),#7321);
#17110=CARTESIAN_POINT ( 'NONE',  ( 103.4083388212532810, 155.0000000000000000, -32.00000000000002842 ) ) ;
#17117=AXIS2_PLACEMENT_3D ( 'NONE', #26039, #12754, #15802 ) ;
#17139=LINE ( 'NONE', #20033, #13693 ) ;
#17167=CYLINDRICAL_SURFACE ( 'NONE', #19990, 31.00000000000000000 ) ;
#17186=DIRECTION ( 'NONE',  ( 0.9945218953682661844, 0.000000000000000000, -0.1045284632677211112 ) ) ;
#17208=VERTEX_POINT ( 'NONE', #8943 ) ;
#17211=DIRECTION ( 'NONE',  ( 1.000000000000000000, -0.000000000000000000, -0.000000000000000000 ) ) ;
#17215=FILL_AREA_STYLE_COLOUR ( '', #4568 ) ;
#17235=CARTESIAN_POINT ( 'NONE',  ( 103.4083388212532810, 155.0000000000000000, 32.00000000000002842 ) ) ;
#17258=DIRECTION ( 'NONE',  ( -0.1045284632676463932, 0.000000000000000000, 0.9945218953682741780 ) ) ;
#17260=CARTESIAN_POINT ( 'NONE',  ( 94.70964751525852421, 155.0000000000000000, 0.000000000000000000 ) ) ;
#17270=VERTEX_POINT ( 'NONE', #19333 ) ;
#17283=CARTESIAN_POINT ( 'NONE',  ( 111.1125082318798007, 155.0000000000000000, 0.000000000000000000 ) ) ;
#17290=VERTEX_POINT ( 'NONE', #26828 ) ;
#17299=VERTEX_POINT ( 'NONE', #29559 ) ;
#17304=DIRECTION ( 'NONE',  ( 0.9945218953682719576, 0.000000000000000000, -0.1045284632676662384 ) ) ;
#17326=FACE_OUTER_BOUND ( 'NONE', #14897, .T. ) ;
#17344=AXIS2_PLACEMENT_3D ( 'NONE', #3259, #5978, #24041 ) ;
#17351=AXIS2_PLACEMENT_3D ( 'NONE', #1724, #10092, #1564 ) ;
#17368=CIRCLE ( 'NONE', #1579, 12.10452846326767684 ) ;
#17374=VERTEX_POINT ( 'NONE', #16601 ) ;
#17377=CARTESIAN_POINT ( 'NONE',  ( 108.1100194822685836, 155.0000000000000000, 13.00000000000003908 ) ) ;
#17378=ORIENTED_EDGE ( 'NONE', *, *, #15438, .T. ) ;
#17380=CYLINDRICAL_SURFACE ( 'NONE', #15616, 31.00000000000000000 ) ;
#17383=ORIENTED_EDGE ( 'NONE', *, *, #23038, .F. ) ;
#17387=VECTOR ( 'NONE', #28132, 1000.000000000000000 ) ;
#17404=ORIENTED_EDGE ( 'NONE', *, *, #7089, .T. ) ;
#17410=ORIENTED_EDGE ( 'NONE', *, *, #32838, .T. ) ;
#17415=CARTESIAN_POINT ( 'NONE',  ( 90.49452189536829394, 155.0000000000000000, 0.000000000000000000 ) ) ;
#17453=CARTESIAN_POINT ( 'NONE',  ( 94.70964751525852421, 155.0000000000000000, -32.10452846326766974 ) ) ;
#17471=EDGE_CURVE ( 'NONE', #25247, #26344, #26264, .T. ) ;
#17506=CARTESIAN_POINT ( 'NONE',  ( 92.60208470531341618, 155.0000000000000000, 0.000000000000000000 ) ) ;
#17512=EDGE_CURVE ( 'NONE', #6439, #20904, #14289, .T. ) ;
#17521=DIRECTION ( 'NONE',  ( -0.1045284632676344722, 0.000000000000000000, 0.9945218953682752883 ) ) ;
#17526=FACE_OUTER_BOUND ( 'NONE', #3149, .T. ) ;
#17569=LINE ( 'NONE', #15354, #12481 ) ;
#17582=ORIENTED_EDGE ( 'NONE', *, *, #27856, .T. ) ;
#17605=SHAPE_REPRESENTATION ( 'High-Force Belleville Spring Washer Pack', ( #2404 ), #30714 ) ;
#17635=EDGE_LOOP ( 'NONE', ( #32241, #10560, #29688, #20438 ) ) ;
#17646=LINE ( 'NONE', #30255, #2313 ) ;
#17663=DIRECTION ( 'NONE',  ( 1.000000000000000000, -0.000000000000000000, -0.000000000000000000 ) ) ;
#17708=CARTESIAN_POINT ( 'NONE',  ( 92.60208470531341618, 155.0000000000000000, 0.000000000000000000 ) ) ;
#17786=VECTOR ( 'NONE', #21271, 1000.000000000000000 ) ;
#17799=EDGE_CURVE ( 'NONE', #22995, #24364, #6659, .T. ) ;
#17861=DIRECTION ( 'NONE',  ( 1.000000000000000000, -0.000000000000000000, -0.000000000000000000 ) ) ;
#17866=ADVANCED_FACE ( 'NONE', ( #10805 ), #18677, .T. ) ;
#17884=CIRCLE ( 'NONE', #8093, 12.00000000000001066 ) ;
#17885=ORIENTED_EDGE ( 'NONE', *, *, #31076, .F. ) ;
#17887=CYLINDRICAL_SURFACE ( 'NONE', #22204, 12.10452846326763598 ) ;
#17892=CARTESIAN_POINT ( 'NONE',  ( 103.3032345859876102, 155.0000000000000000, 0.000000000000000000 ) ) ;
#17920=CARTESIAN_POINT ( 'NONE',  ( 90.49452189536829394, 155.0000000000000000, 32.10452846326766974 ) ) ;
#17984=CARTESIAN_POINT ( 'NONE',  ( 92.60208470531341618, 155.0000000000000000, 0.000000000000000000 ) ) ;
#17990=DIRECTION ( 'NONE',  ( 1.000000000000000000, -0.000000000000000000, -0.000000000000000000 ) ) ;
#18013=ORIENTED_EDGE ( 'NONE', *, *, #31380, .F. ) ;
#18016=DIRECTION ( 'NONE',  ( 0.000000000000000000, 0.000000000000000000, -1.000000000000000000 ) ) ;
#18047=ORIENTED_EDGE ( 'NONE', *, *, #8147, .T. ) ;
#18054=VERTEX_POINT ( 'NONE', #29020 ) ;
#18068=DIRECTION ( 'NONE',  ( -0.1045284632676344722, 1.217938055844717366E-16, -0.9945218953682752883 ) ) ;
#18090=EDGE_CURVE ( 'NONE', #17374, #17299, #14183, .T. ) ;
#18137=ADVANCED_FACE ( 'NONE', ( #16732 ), #13227, .F. ) ;
#18143=EDGE_CURVE ( 'NONE', #11140, #210, #18630, .T. ) ;
#18147=ORIENTED_EDGE ( 'NONE', *, *, #13554, .F. ) ;
#18193=CIRCLE ( 'NONE', #3490, 31.00000000000000000 ) ;
#18217=CARTESIAN_POINT ( 'NONE',  ( 100.2066581602377653, 155.0000000000000000, 13.00000000000001066 ) ) ;
#18222=ORIENTED_EDGE ( 'NONE', *, *, #2730, .F. ) ;
#18239=CARTESIAN_POINT ( 'NONE',  ( 97.30927364589244632, 155.0000000000000000, -31.00000000000000000 ) ) ;
#18258=ORIENTED_EDGE ( 'NONE', *, *, #16025, .F. ) ;
#18260=ORIENTED_EDGE ( 'NONE', *, *, #21976, .T. ) ;
#18283=CARTESIAN_POINT ( 'NONE',  ( 91.60208470531341618, 155.0000000000000000, 12.00000000000001066 ) ) ;
#18291=EDGE_CURVE ( 'NONE', #19123, #21804, #14315, .T. ) ;
#18296=DIRECTION ( 'NONE',  ( 1.000000000000000000, -0.000000000000000000, -0.000000000000000000 ) ) ;
#18301=AXIS2_PLACEMENT_3D ( 'NONE', #32259, #14539, #30221 ) ;
#18330=CARTESIAN_POINT ( 'NONE',  ( 109.0104235265664272, 155.0000000000000000, 0.000000000000000000 ) ) ;
#18388=FACE_OUTER_BOUND ( 'NONE', #1705, .T. ) ;
#18420=EDGE_LOOP ( 'NONE', ( #29736, #31084, #13374, #899 ) ) ;
#18426=CIRCLE ( 'NONE', #24399, 12.00000000000001066 ) ;
#18428=ORIENTED_EDGE ( 'NONE', *, *, #31380, .T. ) ;
#18476=ORIENTED_EDGE ( 'NONE', *, *, #8294, .F. ) ;
#18499=ADVANCED_FACE ( 'NONE', ( #31941 ), #15398, .F. ) ;
#18522=EDGE_CURVE ( 'NONE', #21262, #20010, #3661, .T. ) ;
#18584=DIRECTION ( 'NONE',  ( 0.000000000000000000, 0.000000000000000000, -1.000000000000000000 ) ) ;
#18598=VECTOR ( 'NONE', #26119, 1000.000000000000000 ) ;
#18606=DIRECTION ( 'NONE',  ( 0.000000000000000000, 0.000000000000000000, 1.000000000000000000 ) ) ;
#18622=DIRECTION ( 'NONE',  ( 0.000000000000000000, 0.000000000000000000, -1.000000000000000000 ) ) ;
#18624=LINE ( 'NONE', #26954, #26313 ) ;
#18630=LINE ( 'NONE', #11138, #22462 ) ;
#18639=DIRECTION ( 'NONE',  ( 0.000000000000000000, 0.000000000000000000, -1.000000000000000000 ) ) ;
#18664=VECTOR ( 'NONE', #5072, 1000.000000000000000 ) ;
#18667=CARTESIAN_POINT ( 'NONE',  ( 92.60208470531341618, 155.0000000000000000, 0.000000000000000000 ) ) ;
#18677=CONICAL_SURFACE ( 'NONE', #1263, 32.00000000000000000, 0.1047197551197016768 ) ;
#18682=FACE_OUTER_BOUND ( 'NONE', #21486, .T. ) ;
#18695=EDGE_CURVE ( 'NONE', #17290, #27125, #12683, .T. ) ;
#18714=EDGE_CURVE ( 'NONE', #17208, #23288, #10139, .T. ) ;
#18717=EDGE_LOOP ( 'NONE', ( #11430, #5407, #21551, #19796 ) ) ;
#18734=DIRECTION ( 'NONE',  ( 0.000000000000000000, 0.000000000000000000, -1.000000000000000000 ) ) ;
#18751=CONICAL_SURFACE ( 'NONE', #4049, 32.10452846326766974, 1.466076571675243301 ) ;
#18779=CARTESIAN_POINT ( 'NONE',  ( 105.0134430565187387, 155.0000000000000000, -31.00000000000000000 ) ) ;
#18790=FACE_OUTER_BOUND ( 'NONE', #21141, .T. ) ;
#18805=CARTESIAN_POINT ( 'NONE',  ( 90.49452189536829394, 155.0000000000000000, -32.10452846326766974 ) ) ;
#18835=DIRECTION ( 'NONE',  ( 1.000000000000000000, -0.000000000000000000, -0.000000000000000000 ) ) ;
#18840=CARTESIAN_POINT ( 'NONE',  ( 89.50000000000002842, 155.0000000000000000, 32.00000000000002842 ) ) ;
#18847=CIRCLE ( 'NONE', #8514, 32.10452846326764131 ) ;
#18855=DIRECTION ( 'NONE',  ( 1.000000000000000000, -0.000000000000000000, -0.000000000000000000 ) ) ;
#18868=CONICAL_SURFACE ( 'NONE', #4179, 12.00000000000001066, 0.1047197551196464710 ) ;
#18873=ORIENTED_EDGE ( 'NONE', *, *, #29067, .F. ) ;
#18920=AXIS2_PLACEMENT_3D ( 'NONE', #27585, #4603, #19923 ) ;
#18924=ORIENTED_EDGE ( 'NONE', *, *, #30201, .T. ) ;
#18931=EDGE_LOOP ( 'NONE', ( #29514, #8003, #19170, #10677 ) ) ;
#18934=DIRECTION ( 'NONE',  ( 1.000000000000000000, -0.000000000000000000, -0.000000000000000000 ) ) ;
#18935=CYLINDRICAL_SURFACE ( 'NONE', #17344, 32.00000000000001421 ) ;
#18995=AXIS2_PLACEMENT_3D ( 'NONE', #26156, #23605, #23100 ) ;
#19068=FACE_OUTER_BOUND ( 'NONE', #33355, .T. ) ;
#19078=VECTOR ( 'NONE', #29447, 1000.000000000000000 ) ;
#19080=ORIENTED_EDGE ( 'NONE', *, *, #7911, .T. ) ;
#19123=VERTEX_POINT ( 'NONE', #32405 ) ;
#19149=AXIS2_PLACEMENT_3D ( 'NONE', #21569, #13736, #8305 ) ;
#19167=ORIENTED_EDGE ( 'NONE', *, *, #28298, .F. ) ;
#19170=ORIENTED_EDGE ( 'NONE', *, *, #25408, .F. ) ;
#19179=AXIS2_PLACEMENT_3D ( 'NONE', #17283, #14895, #16938 ) ;
#19233=AXIS2_PLACEMENT_3D ( 'NONE', #25583, #10433, #2248 ) ;
#19256=VECTOR ( 'NONE', #6087, 1000.000000000000000 ) ;
#19268=DIRECTION ( 'NONE',  ( -1.000000000000000000, 0.000000000000000000, 0.000000000000000000 ) ) ;
#19290=CARTESIAN_POINT ( 'NONE',  ( 92.50248874961125978, 155.0000000000000000, 13.00000000000001066 ) ) ;
#19314=LINE ( 'NONE', #10697, #1150 ) ;
#19316=DIRECTION ( 'NONE',  ( 1.000000000000000000, -0.000000000000000000, -0.000000000000000000 ) ) ;
#19318=EDGE_CURVE ( 'NONE', #33225, #31608, #30715, .T. ) ;
#19333=CARTESIAN_POINT ( 'NONE',  ( 108.0159016311981759, 155.0000000000000000, 12.10452846326767684 ) ) ;
#19340=ORIENTED_EDGE ( 'NONE', *, *, #33487, .F. ) ;
#19361=DIRECTION ( 'NONE',  ( 0.000000000000000000, 0.000000000000000000, -1.000000000000000000 ) ) ;
#19374=ORIENTED_EDGE ( 'NONE', *, *, #7292, .F. ) ;
#19378=VECTOR ( 'NONE', #32398, 1000.000000000000114 ) ;
#19439=CIRCLE ( 'NONE', #6944, 32.00000000000002842 ) ;
#19447=EDGE_CURVE ( 'NONE', #8252, #26926, #5085, .T. ) ;
#19462=DIRECTION ( 'NONE',  ( 1.000000000000000000, -0.000000000000000000, -0.000000000000000000 ) ) ;
#19467=VERTEX_POINT ( 'NONE', #7198 ) ;
#19469=CARTESIAN_POINT ( 'NONE',  ( 97.20416941062678973, 155.0000000000000000, 0.000000000000000000 ) ) ;
#19499=ORIENTED_EDGE ( 'NONE', *, *, #23497, .F. ) ;
#19536=DIRECTION ( 'NONE',  ( 1.000000000000000000, -0.000000000000000000, -0.000000000000000000 ) ) ;
#19551=CIRCLE ( 'NONE', #28272, 32.00000000000000000 ) ;
#19558=EDGE_CURVE ( 'NONE', #26344, #25247, #23059, .T. ) ;
#19601=CARTESIAN_POINT ( 'NONE',  ( 102.4138169258850581, 155.0000000000000000, 32.10452846326769816 ) ) ;
#19617=CARTESIAN_POINT ( 'NONE',  ( 100.3117322205716420, 155.0000000000000000, 0.000000000000000000 ) ) ;
#19629=DIRECTION ( 'NONE',  ( 0.000000000000000000, 0.000000000000000000, -1.000000000000000000 ) ) ;
#19656=DIRECTION ( 'NONE',  ( 1.000000000000000000, -0.000000000000000000, -0.000000000000000000 ) ) ;
#19662=CIRCLE ( 'NONE', #29453, 32.10452846326766974 ) ;
#19707=ORIENTED_EDGE ( 'NONE', *, *, #33460, .T. ) ;
#19725=PRODUCT_DEFINITION_FORMATION_WITH_SPECIFIED_SOURCE ( 'ANY', '', #33103, .NOT_KNOWN. ) ;
#19796=ORIENTED_EDGE ( 'NONE', *, *, #23975, .F. ) ;
#19799=EDGE_CURVE ( 'NONE', #29530, #25373, #32198, .T. ) ;
#19830=ORIENTED_EDGE ( 'NONE', *, *, #14588, .F. ) ;
#19850=CYLINDRICAL_SURFACE ( 'NONE', #21595, 13.00000000000002487 ) ;
#19900=DIRECTION ( 'NONE',  ( 0.000000000000000000, 0.000000000000000000, -1.000000000000000000 ) ) ;
#19923=DIRECTION ( 'NONE',  ( 0.000000000000000000, 0.000000000000000000, -1.000000000000000000 ) ) ;
#19947=CARTESIAN_POINT ( 'NONE',  ( 105.9028607166213192, 155.0000000000000000, 0.000000000000000000 ) ) ;
#19967=CIRCLE ( 'NONE', #5284, 12.10452846326767684 ) ;
#19990=AXIS2_PLACEMENT_3D ( 'NONE', #17506, #30463, #4216 ) ;
#19998=VECTOR ( 'NONE', #25441, 1000.000000000000114 ) ;
#20010=VERTEX_POINT ( 'NONE', #17377 ) ;
#20033=CARTESIAN_POINT ( 'NONE',  ( 95.59906517536109050, 155.0000000000000000, 31.00000000000000000 ) ) ;
#20091=VECTOR ( 'NONE', #22515, 1000.000000000000227 ) ;
#20094=CARTESIAN_POINT ( 'NONE',  ( 108.0159016311981759, 155.0000000000000000, -12.10452846326767684 ) ) ;
#20160=CARTESIAN_POINT ( 'NONE',  ( 92.60208470531341618, 155.0000000000000000, 12.99999999999999822 ) ) ;
#20212=FACE_OUTER_BOUND ( 'NONE', #18717, .T. ) ;
#20219=VECTOR ( 'NONE', #1216, 1000.000000000000000 ) ;
#20242=CARTESIAN_POINT ( 'NONE',  ( 109.0104235265664272, 155.0000000000000000, 0.000000000000000000 ) ) ;
#20264=DIRECTION ( 'NONE',  ( 1.000000000000000000, -0.000000000000000000, -0.000000000000000000 ) ) ;
#20293=CONICAL_SURFACE ( 'NONE', #32248, 32.00000000000000000, 0.1047197551197278087 ) ;
#20346=ORIENTED_EDGE ( 'NONE', *, *, #7239, .T. ) ;
#20406=EDGE_CURVE ( 'NONE', #24364, #31583, #21598, .T. ) ;
#20416=CARTESIAN_POINT ( 'NONE',  ( 92.60208470531341618, 155.0000000000000000, -12.10452846326765020 ) ) ;
#20421=DIRECTION ( 'NONE',  ( 0.000000000000000000, 0.000000000000000000, 1.000000000000000000 ) ) ;
#20427=CARTESIAN_POINT ( 'NONE',  ( 100.3007760113082156, 155.0000000000000000, 0.000000000000000000 ) ) ;
#20431=VERTEX_POINT ( 'NONE', #3713 ) ;
#20438=ORIENTED_EDGE ( 'NONE', *, *, #3445, .F. ) ;
#20439=ORIENTED_EDGE ( 'NONE', *, *, #16025, .T. ) ;
#20442=ORIENTED_EDGE ( 'NONE', *, *, #2735, .T. ) ;
#20448=ORIENTED_EDGE ( 'NONE', *, *, #10868, .T. ) ;
#20479=ORIENTED_EDGE ( 'NONE', *, *, #23497, .T. ) ;
#20496=DIRECTION ( 'NONE',  ( 0.000000000000000000, 0.000000000000000000, -1.000000000000000000 ) ) ;
#20526=VERTEX_POINT ( 'NONE', #24160 ) ;
#20534=AXIS2_PLACEMENT_3D ( 'NONE', #12726, #7284, #25497 ) ;
#20538=AXIS2_PLACEMENT_3D ( 'NONE', #32423, #3982, #11318 ) ;
#20553=DIRECTION ( 'NONE',  ( 0.000000000000000000, 0.000000000000000000, -1.000000000000000000 ) ) ;
#20557=CONICAL_SURFACE ( 'NONE', #29258, 12.00000000000001066, 0.1047197551196174109 ) ;
#20568=CONICAL_SURFACE ( 'NONE', #30916, 11.99999999999998224, 0.1047197551196726167 ) ;
#20571=CARTESIAN_POINT ( 'NONE',  ( 111.1125082318798007, 155.0000000000000000, 32.00000000000002842 ) ) ;
#20579=LINE ( 'NONE', #30984, #18664 ) ;
#20614=AXIS2_PLACEMENT_3D ( 'NONE', #31950, #13896, #20906 ) ;
#20658=DIRECTION ( 'NONE',  ( 0.000000000000000000, 0.000000000000000000, -1.000000000000000000 ) ) ;
#20662=AXIS2_PLACEMENT_3D ( 'NONE', #31850, #13460, #18584 ) ;
#20675=CARTESIAN_POINT ( 'NONE',  ( 111.1125082318798007, 155.0000000000000000, 32.00000000000002842 ) ) ;
#20677=CARTESIAN_POINT ( 'NONE',  ( 104.9083388212530537, 155.0000000000000000, 0.000000000000000000 ) ) ;
#20710=AXIS2_PLACEMENT_3D ( 'NONE', #9174, #4219, #24840 ) ;
#20756=DIRECTION ( 'NONE',  ( 0.000000000000000000, 0.000000000000000000, -1.000000000000000000 ) ) ;
#20766=ORIENTED_EDGE ( 'NONE', *, *, #14716, .F. ) ;
#20778=ORIENTED_EDGE ( 'NONE', *, *, #19447, .T. ) ;
#20789=VECTOR ( 'NONE', #16799, 1000.000000000000000 ) ;
#20860=ORIENTED_EDGE ( 'NONE', *, *, #978, .F. ) ;
#20874=CONICAL_SURFACE ( 'NONE', #26839, 32.00000000000002842, 0.1047197551196464710 ) ;
#20882=CARTESIAN_POINT ( 'NONE',  ( 100.4058500716420781, 155.0000000000000000, 12.99999999999998401 ) ) ;
#20904=VERTEX_POINT ( 'NONE', #20571 ) ;
#20906=DIRECTION ( 'NONE',  ( 0.000000000000000000, 0.000000000000000000, 1.000000000000000000 ) ) ;
#20951=( LENGTH_UNIT ( ) NAMED_UNIT ( * ) SI_UNIT ( .MILLI., .METRE. ) );
#20964=ADVANCED_FACE ( 'NONE', ( #32757 ), #10024, .T. ) ;
#20981=DIRECTION ( 'NONE',  ( 1.000000000000000000, -0.000000000000000000, -0.000000000000000000 ) ) ;
#20994=CARTESIAN_POINT ( 'NONE',  ( 100.3007760113082156, 155.0000000000000000, 0.000000000000000000 ) ) ;
#21030=CARTESIAN_POINT ( 'NONE',  ( 103.3032345859876102, 155.0000000000000000, 31.00000000000000000 ) ) ;
#21035=DIRECTION ( 'NONE',  ( 1.000000000000000000, -0.000000000000000000, -0.000000000000000000 ) ) ;
#21061=ORIENTED_EDGE ( 'NONE', *, *, #27422, .F. ) ;
#21080=CARTESIAN_POINT ( 'NONE',  ( 108.1100194822685836, 155.0000000000000000, 0.000000000000000000 ) ) ;
#21081=CARTESIAN_POINT ( 'NONE',  ( 94.70964751525852421, 155.0000000000000000, 0.000000000000000000 ) ) ;
#21117=( LENGTH_UNIT ( ) NAMED_UNIT ( * ) SI_UNIT ( .MILLI., .METRE. ) );
#21120=VECTOR ( 'NONE', #12242, 1000.000000000000000 ) ;
#21141=EDGE_LOOP ( 'NONE', ( #27339, #3652, #13337, #18873 ) ) ;
#21152=DIRECTION ( 'NONE',  ( 1.000000000000000000, -0.000000000000000000, -0.000000000000000000 ) ) ;
#21154=VECTOR ( 'NONE', #3308, 1000.000000000000000 ) ;
#21157=CARTESIAN_POINT ( 'NONE',  ( 105.9028607166213192, 155.0000000000000000, 32.10452846326769816 ) ) ;
#21173=EDGE_CURVE ( 'NONE', #29217, #19467, #31187, .T. ) ;
#21189=CARTESIAN_POINT ( 'NONE',  ( 95.59906517536109050, 155.0000000000000000, 0.000000000000000000 ) ) ;
#21205=ORIENTED_EDGE ( 'NONE', *, *, #3537, .F. ) ;
#21206=DIRECTION ( 'NONE',  ( 1.000000000000000000, -0.000000000000000000, -0.000000000000000000 ) ) ;
#21242=ADVANCED_FACE ( 'NONE', ( #18682 ), #29543, .T. ) ;
#21262=VERTEX_POINT ( 'NONE', #6528 ) ;
#21264=AXIS2_PLACEMENT_3D ( 'NONE', #16326, #13774, #16663 ) ;
#21271=DIRECTION ( 'NONE',  ( -0.1045284632676468234, 1.217938055844715641E-16, -0.9945218953682740670 ) ) ;
#21347=ORIENTED_EDGE ( 'NONE', *, *, #22652, .F. ) ;
#21374=DIRECTION ( 'NONE',  ( 1.000000000000000000, -0.000000000000000000, -0.000000000000000000 ) ) ;
#21401=DIRECTION ( 'NONE',  ( -0.9945218953682687379, 1.280104479605762779E-17, -0.1045284632676965614 ) ) ;
#21429=VERTEX_POINT ( 'NONE', #33091 ) ;
#21473=ADVANCED_FACE ( 'NONE', ( #14035 ), #881, .F. ) ;
#21486=EDGE_LOOP ( 'NONE', ( #123, #23504, #32583, #22828 ) ) ;
#21518=ORIENTED_EDGE ( 'NONE', *, *, #2040, .T. ) ;
#21525=CARTESIAN_POINT ( 'NONE',  ( 107.9108275708642850, 155.0000000000000000, 0.000000000000000000 ) ) ;
#21551=ORIENTED_EDGE ( 'NONE', *, *, #2095, .T. ) ;
#21561=AXIS2_PLACEMENT_3D ( 'NONE', #5051, #16063, #31895 ) ;
#21569=CARTESIAN_POINT ( 'NONE',  ( 95.70416941062676131, 155.0000000000000000, 0.000000000000000000 ) ) ;
#21582=AXIS2_PLACEMENT_3D ( 'NONE', #5977, #18934, #16364 ) ;
#21584=EDGE_CURVE ( 'NONE', #19123, #1694, #9598, .T. ) ;
#21586=CIRCLE ( 'NONE', #5282, 12.00000000000001066 ) ;
#21595=AXIS2_PLACEMENT_3D ( 'NONE', #4350, #24460, #3670 ) ;
#21598=LINE ( 'NONE', #10893, #19256 ) ;
#21605=( NAMED_UNIT ( * ) PLANE_ANGLE_UNIT ( ) SI_UNIT ( $, .RADIAN. ) );
#21625=AXIS2_PLACEMENT_3D ( 'NONE', #5037, #21035, #424 ) ;
#21663=DIRECTION ( 'NONE',  ( 1.000000000000000000, -0.000000000000000000, -0.000000000000000000 ) ) ;
#21683=DIRECTION ( 'NONE',  ( -0.9945218953682772867, 0.000000000000000000, 0.1045284632676156678 ) ) ;
#21685=ORIENTED_EDGE ( 'NONE', *, *, #13698, .F. ) ;
#21693=ORIENTED_EDGE ( 'NONE', *, *, #21584, .F. ) ;
#21711=CIRCLE ( 'NONE', #5378, 32.10452846326769816 ) ;
#21714=ORIENTED_EDGE ( 'NONE', *, *, #16249, .F. ) ;
#21765=CARTESIAN_POINT ( 'NONE',  ( 107.0104235265664556, 155.0000000000000000, 0.000000000000000000 ) ) ;
#21772=ORIENTED_EDGE ( 'NONE', *, *, #28569, .T. ) ;
#21776=FACE_OUTER_BOUND ( 'NONE', #26306, .T. ) ;
#21804=VERTEX_POINT ( 'NONE', #22209 ) ;
#21833=ORIENTED_EDGE ( 'NONE', *, *, #6430, .T. ) ;
#21865=DIRECTION ( 'NONE',  ( 1.000000000000000000, -0.000000000000000000, -0.000000000000000000 ) ) ;
#21869=VERTEX_POINT ( 'NONE', #4664 ) ;
#21871=AXIS2_PLACEMENT_3D ( 'NONE', #16457, #5733, #13908 ) ;
#21885=ADVANCED_FACE ( 'NONE', ( #25788 ), #31075, .F. ) ;
#21919=CIRCLE ( 'NONE', #6708, 13.00000000000001066 ) ;
#21969=EDGE_LOOP ( 'NONE', ( #14304, #27374, #8652, #18924 ) ) ;
#21976=EDGE_CURVE ( 'NONE', #82, #30802, #25947, .T. ) ;
#21980=CARTESIAN_POINT ( 'NONE',  ( 92.60208470531341618, 155.0000000000000000, -13.00000000000002487 ) ) ;
#21992=LINE ( 'NONE', #5809, #3753 ) ;
#22003=CARTESIAN_POINT ( 'NONE',  ( 90.49452189536829394, 155.0000000000000000, 0.000000000000000000 ) ) ;
#22010=CARTESIAN_POINT ( 'NONE',  ( 97.20416941062678973, 155.0000000000000000, -32.00000000000000000 ) ) ;
#22029=CARTESIAN_POINT ( 'NONE',  ( 109.0104235265664272, 155.0000000000000000, 0.000000000000000000 ) ) ;
#22045=ORIENTED_EDGE ( 'NONE', *, *, #4396, .T. ) ;
#22147=VECTOR ( 'NONE', #24794, 1000.000000000000227 ) ;
#22196=CARTESIAN_POINT ( 'NONE',  ( 103.4083388212532810, 155.0000000000000000, 0.000000000000000000 ) ) ;
#22204=AXIS2_PLACEMENT_3D ( 'NONE', #28781, #20264, #31014 ) ;
#22209=CARTESIAN_POINT ( 'NONE',  ( 99.30625411593993590, 155.0000000000000000, -12.00000000000001066 ) ) ;
#22210=AXIS2_PLACEMENT_3D ( 'NONE', #14456, #24852, #11912 ) ;
#22247=AXIS2_PLACEMENT_3D ( 'NONE', #12608, #17211, #27440 ) ;
#22279=ADVANCED_FACE ( 'NONE', ( #10171 ), #25393, .T. ) ;
#22316=ORIENTED_EDGE ( 'NONE', *, *, #7714, .T. ) ;
#22321=ORIENTED_EDGE ( 'NONE', *, *, #25562, .T. ) ;
#22365=CARTESIAN_POINT ( 'NONE',  ( 103.3032345859876102, 155.0000000000000000, -31.00000000000000000 ) ) ;
#22373=DIRECTION ( 'NONE',  ( 0.9945218953682777308, 1.280104479604719079E-17, 0.1045284632676113518 ) ) ;
#22388=DIRECTION ( 'NONE',  ( 1.000000000000000000, -0.000000000000000000, -0.000000000000000000 ) ) ;
#22394=DIRECTION ( 'NONE',  ( 0.000000000000000000, 0.000000000000000000, -1.000000000000000000 ) ) ;
#22430=EDGE_LOOP ( 'NONE', ( #5968, #2384, #6014, #12257 ) ) ;
#22443=EDGE_CURVE ( 'NONE', #19467, #17270, #3117, .T. ) ;
#22462=VECTOR ( 'NONE', #29184, 1000.000000000000000 ) ;
#22477=CARTESIAN_POINT ( 'NONE',  ( 91.60208470531341618, 155.0000000000000000, 0.000000000000000000 ) ) ;
#22481=ADVANCED_FACE ( 'NONE', ( #24573 ), #4293, .T. ) ;
#22502=PRESENTATION_STYLE_ASSIGNMENT (( #12111 ) ) ;
#22515=DIRECTION ( 'NONE',  ( 0.9945218953682719576, 1.280104479605391614E-17, 0.1045284632676662384 ) ) ;
#22522=VECTOR ( 'NONE', #8858, 1000.000000000000000 ) ;
#22538=ORIENTED_EDGE ( 'NONE', *, *, #27673, .F. ) ;
#22652=EDGE_CURVE ( 'NONE', #9110, #6991, #25929, .T. ) ;
#22654=ORIENTED_EDGE ( 'NONE', *, *, #25009, .F. ) ;
#22705=VECTOR ( 'NONE', #31239, 1000.000000000000000 ) ;
#22749=VERTEX_POINT ( 'NONE', #7705 ) ;
#22762=DIRECTION ( 'NONE',  ( 0.000000000000000000, 0.000000000000000000, -1.000000000000000000 ) ) ;
#22780=CONICAL_SURFACE ( 'NONE', #22210, 32.00000000000002842, 0.1047197551196217685 ) ;
#22792=DIRECTION ( 'NONE',  ( 0.1045284632676459352, 1.217938055844715641E-16, 0.9945218953682740670 ) ) ;
#22812=CARTESIAN_POINT ( 'NONE',  ( 104.9083388212530537, 155.0000000000000000, -32.00000000000000000 ) ) ;
#22822=DIRECTION ( 'NONE',  ( 0.000000000000000000, 0.000000000000000000, -1.000000000000000000 ) ) ;
#22828=ORIENTED_EDGE ( 'NONE', *, *, #32504, .F. ) ;
#22849=DIRECTION ( 'NONE',  ( -1.000000000000000000, 0.000000000000000000, 0.000000000000000000 ) ) ;
#22862=ORIENTED_EDGE ( 'NONE', *, *, #19558, .F. ) ;
#22875=ORIENTED_EDGE ( 'NONE', *, *, #31845, .F. ) ;
#22916=ORIENTED_EDGE ( 'NONE', *, *, #23137, .T. ) ;
#22943=DIRECTION ( 'NONE',  ( 1.000000000000000000, -0.000000000000000000, -0.000000000000000000 ) ) ;
#22959=ORIENTED_EDGE ( 'NONE', *, *, #4396, .F. ) ;
#22960=CARTESIAN_POINT ( 'NONE',  ( 92.60208470531341618, 155.0000000000000000, 32.00000000000001421 ) ) ;
#22980=AXIS2_PLACEMENT_3D ( 'NONE', #32046, #8218, #5486 ) ;
#22986=CARTESIAN_POINT ( 'NONE',  ( 104.9083388212530537, 155.0000000000000000, 0.000000000000000000 ) ) ;
#22995=VERTEX_POINT ( 'NONE', #16350 ) ;
#23003=AXIS2_PLACEMENT_3D ( 'NONE', #23068, #8079, #10472 ) ;
#23018=CARTESIAN_POINT ( 'NONE',  ( 98.19869130599479945, 155.0000000000000000, 0.000000000000000000 ) ) ;
#23038=EDGE_CURVE ( 'NONE', #14731, #28067, #13802, .T. ) ;
#23046=VECTOR ( 'NONE', #15139, 1000.000000000000000 ) ;
#23059=CIRCLE ( 'NONE', #2368, 32.00000000000002842 ) ;
#23060=DIRECTION ( 'NONE',  ( 0.000000000000000000, 0.000000000000000000, -1.000000000000000000 ) ) ;
#23068=CARTESIAN_POINT ( 'NONE',  ( 92.70168066101555837, 155.0000000000000000, 0.000000000000000000 ) ) ;
#23072=DIRECTION ( 'NONE',  ( 1.000000000000000000, -0.000000000000000000, -0.000000000000000000 ) ) ;
#23079=ORIENTED_EDGE ( 'NONE', *, *, #23649, .T. ) ;
#23087=CARTESIAN_POINT ( 'NONE',  ( 92.70168066101555837, 155.0000000000000000, 13.00000000000003908 ) ) ;
#23100=DIRECTION ( 'NONE',  ( 0.000000000000000000, 0.000000000000000000, -1.000000000000000000 ) ) ;
#23113=CYLINDRICAL_SURFACE ( 'NONE', #8840, 12.99999999999999822 ) ;
#23137=EDGE_CURVE ( 'NONE', #31501, #18054, #2548, .T. ) ;
#23140=EDGE_CURVE ( 'NONE', #17299, #210, #29189, .T. ) ;
#23165=CARTESIAN_POINT ( 'NONE',  ( 89.50000000000002842, 155.0000000000000000, -32.00000000000002842 ) ) ;
#23230=ORIENTED_EDGE ( 'NONE', *, *, #1394, .F. ) ;
#23235=AXIS2_PLACEMENT_3D ( 'NONE', #17708, #2041, #10392 ) ;
#23247=ORIENTED_EDGE ( 'NONE', *, *, #19318, .F. ) ;
#23258=AXIS2_PLACEMENT_3D ( 'NONE', #12551, #22943, #4887 ) ;
#23263=EDGE_CURVE ( 'NONE', #6991, #546, #12428, .T. ) ;
#23285=ORIENTED_EDGE ( 'NONE', *, *, #32696, .T. ) ;
#23288=VERTEX_POINT ( 'NONE', #30663 ) ;
#23296=ADVANCED_FACE ( 'NONE', ( #33032 ), #18868, .F. ) ;
#23326=ADVANCED_FACE ( 'NONE', ( #28276 ), #31411, .T. ) ;
#23342=ADVANCED_FACE ( 'NONE', ( #12256 ), #12769, .F. ) ;
#23367=LINE ( 'NONE', #17920, #17387 ) ;
#23382=VERTEX_POINT ( 'NONE', #20094 ) ;
#23405=VERTEX_POINT ( 'NONE', #18217 ) ;
#23410=ORIENTED_EDGE ( 'NONE', *, *, #32504, .T. ) ;
#23426=AXIS2_PLACEMENT_3D ( 'NONE', #11078, #16169, #13786 ) ;
#23471=DIRECTION ( 'NONE',  ( 1.000000000000000000, -0.000000000000000000, -0.000000000000000000 ) ) ;
#23492=ORIENTED_EDGE ( 'NONE', *, *, #26864, .F. ) ;
#23494=AXIS2_PLACEMENT_3D ( 'NONE', #32306, #1802, #32467 ) ;
#23497=EDGE_CURVE ( 'NONE', #18054, #31501, #21586, .T. ) ;
#23504=ORIENTED_EDGE ( 'NONE', *, *, #13698, .T. ) ;
#23516=CONICAL_SURFACE ( 'NONE', #27853, 32.00000000000002842, 1.466076571675243523 ) ;
#23521=FACE_OUTER_BOUND ( 'NONE', #6610, .T. ) ;
#23558=VECTOR ( 'NONE', #24352, 999.9999999999998863 ) ;
#23570=ORIENTED_EDGE ( 'NONE', *, *, #14716, .T. ) ;
#23580=CARTESIAN_POINT ( 'NONE',  ( 92.59660660068168170, 155.0000000000000000, 0.000000000000000000 ) ) ;
#23596=DIRECTION ( 'NONE',  ( -0.9945218953682717355, 0.000000000000000000, 0.1045284632676676817 ) ) ;
#23605=DIRECTION ( 'NONE',  ( 1.000000000000000000, -0.000000000000000000, -0.000000000000000000 ) ) ;
#23609=DIRECTION ( 'NONE',  ( 0.000000000000000000, 0.000000000000000000, -1.000000000000000000 ) ) ;
#23649=EDGE_CURVE ( 'NONE', #31501, #22995, #16141, .T. ) ;
#23658=VERTEX_POINT ( 'NONE', #26533 ) ;
#23662=DIRECTION ( 'NONE',  ( 1.000000000000000000, -0.000000000000000000, -0.000000000000000000 ) ) ;
#23684=DIRECTION ( 'NONE',  ( 1.000000000000000000, -0.000000000000000000, -0.000000000000000000 ) ) ;
#23689=CARTESIAN_POINT ( 'NONE',  ( 102.4138169258850581, 155.0000000000000000, -32.10452846326769816 ) ) ;
#23698=EDGE_LOOP ( 'NONE', ( #9564, #6823, #29022, #29468 ) ) ;
#23705=ORIENTED_EDGE ( 'NONE', *, *, #17471, .F. ) ;
#23712=FACE_OUTER_BOUND ( 'NONE', #22430, .T. ) ;
#23728=ORIENTED_EDGE ( 'NONE', *, *, #31819, .F. ) ;
#23750=ORIENTED_EDGE ( 'NONE', *, *, #13855, .F. ) ;
#23779=VERTEX_POINT ( 'NONE', #14258 ) ;
#23800=DIRECTION ( 'NONE',  ( 0.000000000000000000, 0.000000000000000000, -1.000000000000000000 ) ) ;
#23871=ADVANCED_FACE ( 'NONE', ( #17326 ), #1485, .T. ) ;
#23947=ORIENTED_EDGE ( 'NONE', *, *, #3537, .T. ) ;
#23949=ORIENTED_EDGE ( 'NONE', *, *, #15294, .T. ) ;
#23952=ORIENTED_EDGE ( 'NONE', *, *, #624, .F. ) ;
#23967=ADVANCED_FACE ( 'NONE', ( #30616 ), #30448, .T. ) ;
#23975=EDGE_CURVE ( 'NONE', #22995, #27125, #4712, .T. ) ;
#23977=EDGE_CURVE ( 'NONE', #4327, #15528, #3667, .T. ) ;
#23987=ORIENTED_EDGE ( 'NONE', *, *, #4342, .T. ) ;
#24027=ORIENTED_EDGE ( 'NONE', *, *, #1411, .F. ) ;
#24039=LINE ( 'NONE', #707, #33315 ) ;
#24041=DIRECTION ( 'NONE',  ( 0.000000000000000000, 0.000000000000000000, -1.000000000000000000 ) ) ;
#24048=CARTESIAN_POINT ( 'NONE',  ( 107.9108275708642850, 155.0000000000000000, 0.000000000000000000 ) ) ;
#24060=DIRECTION ( 'NONE',  ( -1.000000000000000000, 0.000000000000000000, 0.000000000000000000 ) ) ;
#24109=ORIENTED_EDGE ( 'NONE', *, *, #27506, .F. ) ;
#24156=ADVANCED_FACE ( 'NONE', ( #611 ), #6934, .F. ) ;
#24157=EDGE_CURVE ( 'NONE', #28067, #210, #32447, .T. ) ;
#24160=CARTESIAN_POINT ( 'NONE',  ( 98.19869130599479945, 155.0000000000000000, 32.10452846326769816 ) ) ;
#24210=CARTESIAN_POINT ( 'NONE',  ( 92.60208470531341618, 155.0000000000000000, 0.000000000000000000 ) ) ;
#24220=DIRECTION ( 'NONE',  ( 1.000000000000000000, -0.000000000000000000, -0.000000000000000000 ) ) ;
#24234=DIRECTION ( 'NONE',  ( 0.000000000000000000, 0.000000000000000000, 1.000000000000000000 ) ) ;
#24242=FACE_OUTER_BOUND ( 'NONE', #1566, .T. ) ;
#24293=CARTESIAN_POINT ( 'NONE',  ( 92.60756280994512224, 155.0000000000000000, 0.000000000000000000 ) ) ;
#24306=CIRCLE ( 'NONE', #8563, 32.10452846326764131 ) ;
#24311=EDGE_LOOP ( 'NONE', ( #4601, #18047, #6472, #23230 ) ) ;
#24330=LINE ( 'NONE', #21157, #14500 ) ;
#24352=DIRECTION ( 'NONE',  ( 0.1045284632676472814, 0.000000000000000000, -0.9945218953682740670 ) ) ;
#24364=VERTEX_POINT ( 'NONE', #4168 ) ;
#24367=ADVANCED_FACE ( 'NONE', ( #8778 ), #12008, .F. ) ;
#24368=ORIENTED_EDGE ( 'NONE', *, *, #179, .T. ) ;
#24381=DIRECTION ( 'NONE',  ( 0.1045284632676470454, 1.217938055844715641E-16, 0.9945218953682739560 ) ) ;
#24392=LINE ( 'NONE', #13493, #20219 ) ;
#24394=AXIS2_PLACEMENT_3D ( 'NONE', #25311, #1975, #22762 ) ;
#24399=AXIS2_PLACEMENT_3D ( 'NONE', #28614, #9882, #25376 ) ;
#24420=DIRECTION ( 'NONE',  ( 0.000000000000000000, 0.000000000000000000, -1.000000000000000000 ) ) ;
#24432=LINE ( 'NONE', #27157, #27605 ) ;
#24457=ORIENTED_EDGE ( 'NONE', *, *, #10027, .F. ) ;
#24460=DIRECTION ( 'NONE',  ( 1.000000000000000000, -0.000000000000000000, -0.000000000000000000 ) ) ;
#24473=DIRECTION ( 'NONE',  ( 0.1045284632676459352, 1.217938055844715641E-16, 0.9945218953682740670 ) ) ;
#24496=ADVANCED_FACE ( 'NONE', ( #7076 ), #20557, .F. ) ;
#24531=CARTESIAN_POINT ( 'NONE',  ( 90.49452189536829394, 155.0000000000000000, -32.10452846326766974 ) ) ;
#24535=EDGE_LOOP ( 'NONE', ( #24457, #9355, #30787, #14361 ) ) ;
#24573=FACE_OUTER_BOUND ( 'NONE', #31051, .T. ) ;
#24586=DIRECTION ( 'NONE',  ( 1.000000000000000000, -0.000000000000000000, -0.000000000000000000 ) ) ;
#24621=ORIENTED_EDGE ( 'NONE', *, *, #13554, .T. ) ;
#24625=DIRECTION ( 'NONE',  ( 1.000000000000000000, -0.000000000000000000, -0.000000000000000000 ) ) ;
#24631=AXIS2_PLACEMENT_3D ( 'NONE', #28183, #2126, #25797 ) ;
#24668=AXIS2_PLACEMENT_3D ( 'NONE', #20427, #31154, #30820 ) ;
#24746=DIRECTION ( 'NONE',  ( 1.000000000000000000, -0.000000000000000000, -0.000000000000000000 ) ) ;
#24794=DIRECTION ( 'NONE',  ( 0.1045284632676470454, 0.000000000000000000, -0.9945218953682739560 ) ) ;
#24823=EDGE_LOOP ( 'NONE', ( #19340, #22045, #5106, #17885 ) ) ;
#24829=AXIS2_PLACEMENT_3D ( 'NONE', #1912, #6337, #32912 ) ;
#24840=DIRECTION ( 'NONE',  ( 0.000000000000000000, 0.000000000000000000, -1.000000000000000000 ) ) ;
#24852=DIRECTION ( 'NONE',  ( -1.000000000000000000, 0.000000000000000000, 0.000000000000000000 ) ) ;
#24855=DIRECTION ( 'NONE',  ( 0.000000000000000000, 0.000000000000000000, -1.000000000000000000 ) ) ;
#24868=ORIENTED_EDGE ( 'NONE', *, *, #32456, .T. ) ;
#24875=VECTOR ( 'NONE', #32988, 1000.000000000000000 ) ;
#24880=DIRECTION ( 'NONE',  ( -0.1045284632676468234, 0.000000000000000000, 0.9945218953682740670 ) ) ;
#24890=VECTOR ( 'NONE', #19656, 1000.000000000000000 ) ;
#24935=CONICAL_SURFACE ( 'NONE', #33105, 12.00000000000001066, 0.1047197551196464710 ) ;
#24970=DIRECTION ( 'NONE',  ( 1.000000000000000000, -0.000000000000000000, -0.000000000000000000 ) ) ;
#25009=EDGE_CURVE ( 'NONE', #20526, #3157, #8072, .T. ) ;
#25054=CARTESIAN_POINT ( 'NONE',  ( 97.20416941062678973, 155.0000000000000000, 32.00000000000000000 ) ) ;
#25088=FACE_OUTER_BOUND ( 'NONE', #10316, .T. ) ;
#25092=CARTESIAN_POINT ( 'NONE',  ( 105.0134430565187387, 155.0000000000000000, 31.00000000000000000 ) ) ;
#25109=ORIENTED_EDGE ( 'NONE', *, *, #27506, .T. ) ;
#25119=CARTESIAN_POINT ( 'NONE',  ( 99.30625411593993590, 155.0000000000000000, 0.000000000000000000 ) ) ;
#25129=CARTESIAN_POINT ( 'NONE',  ( 92.60208470531341618, 155.0000000000000000, -32.00000000000002842 ) ) ;
#25156=ORIENTED_EDGE ( 'NONE', *, *, #18714, .F. ) ;
#25185=VECTOR ( 'NONE', #32955, 1000.000000000000000 ) ;
#25212=EDGE_CURVE ( 'NONE', #17290, #26453, #18426, .T. ) ;
#25238=FACE_OUTER_BOUND ( 'NONE', #11541, .T. ) ;
#25247=VERTEX_POINT ( 'NONE', #23165 ) ;
#25260=DIRECTION ( 'NONE',  ( -1.000000000000000000, 0.000000000000000000, 0.000000000000000000 ) ) ;
#25283=EDGE_LOOP ( 'NONE', ( #20860, #14766, #18260, #31136 ) ) ;
#25311=CARTESIAN_POINT ( 'NONE',  ( 95.59906517536109050, 155.0000000000000000, 0.000000000000000000 ) ) ;
#25356=ADVANCED_FACE ( 'NONE', ( #18388 ), #17887, .F. ) ;
#25370=CARTESIAN_POINT ( 'NONE',  ( 102.4138169258850581, 155.0000000000000000, 32.10452846326769816 ) ) ;
#25373=VERTEX_POINT ( 'NONE', #29437 ) ;
#25376=DIRECTION ( 'NONE',  ( 0.000000000000000000, 0.000000000000000000, -1.000000000000000000 ) ) ;
#25378=EDGE_LOOP ( 'NONE', ( #16181, #12390, #9788, #14607 ) ) ;
#25393=CONICAL_SURFACE ( 'NONE', #21561, 32.00000000000005684, 0.1047197551196217685 ) ;
#25397=FACE_OUTER_BOUND ( 'NONE', #9156, .T. ) ;
#25408=EDGE_CURVE ( 'NONE', #31608, #12687, #28756, .T. ) ;
#25412=ORIENTED_EDGE ( 'NONE', *, *, #12909, .F. ) ;
#25440=FACE_OUTER_BOUND ( 'NONE', #14819, .T. ) ;
#25441=DIRECTION ( 'NONE',  ( 0.1045284632676459352, 0.000000000000000000, -0.9945218953682740670 ) ) ;
#25451=FACE_OUTER_BOUND ( 'NONE', #14039, .T. ) ;
#25497=DIRECTION ( 'NONE',  ( 0.000000000000000000, 0.000000000000000000, -1.000000000000000000 ) ) ;
#25518=CYLINDRICAL_SURFACE ( 'NONE', #31626, 13.00000000000002487 ) ;
#25554=DIRECTION ( 'NONE',  ( 0.000000000000000000, 0.000000000000000000, -1.000000000000000000 ) ) ;
#25562=EDGE_CURVE ( 'NONE', #20431, #33389, #27649, .T. ) ;
#25583=CARTESIAN_POINT ( 'NONE',  ( 102.4138169258850581, 155.0000000000000000, 0.000000000000000000 ) ) ;
#25587=ADVANCED_FACE ( 'NONE', ( #32155 ), #24935, .F. ) ;
#25627=EDGE_LOOP ( 'NONE', ( #19830, #32231, #10177, #32766 ) ) ;
#25643=CARTESIAN_POINT ( 'NONE',  ( 101.3062541159399075, 155.0000000000000000, 12.00000000000001066 ) ) ;
#25693=FACE_OUTER_BOUND ( 'NONE', #24535, .T. ) ;
#25703=AXIS2_PLACEMENT_3D ( 'NONE', #24293, #26517, #6063 ) ;
#25707=AXIS2_PLACEMENT_3D ( 'NONE', #23580, #18296, #31252 ) ;
#25717=ORIENTED_EDGE ( 'NONE', *, *, #18090, .T. ) ;
#25729=AXIS2_PLACEMENT_3D ( 'NONE', #31737, #8409, #24234 ) ;
#25788=FACE_OUTER_BOUND ( 'NONE', #17635, .T. ) ;
#25797=DIRECTION ( 'NONE',  ( 0.000000000000000000, 0.000000000000000000, 1.000000000000000000 ) ) ;
#25874=CARTESIAN_POINT ( 'NONE',  ( 104.9083388212530537, 155.0000000000000000, 32.00000000000000000 ) ) ;
#25891=CARTESIAN_POINT ( 'NONE',  ( 108.0159016311981759, 155.0000000000000000, 0.000000000000000000 ) ) ;
#25929=CIRCLE ( 'NONE', #24829, 12.99999999999998401 ) ;
#25940=DIRECTION ( 'NONE',  ( 0.000000000000000000, 0.000000000000000000, 1.000000000000000000 ) ) ;
#25941=CIRCLE ( 'NONE', #3080, 12.10452846326762177 ) ;
#25947=LINE ( 'NONE', #33622, #19998 ) ;
#25955=AXIS2_PLACEMENT_3D ( 'NONE', #29052, #21374, #29716 ) ;
#25965=ORIENTED_EDGE ( 'NONE', *, *, #7089, .F. ) ;
#25979=EDGE_CURVE ( 'NONE', #32773, #23288, #10273, .T. ) ;
#25990=CIRCLE ( 'NONE', #20538, 32.00000000000005684 ) ;
#26006=AXIS2_PLACEMENT_3D ( 'NONE', #21189, #26466, #18639 ) ;
#26020=DIRECTION ( 'NONE',  ( 0.000000000000000000, 0.000000000000000000, -1.000000000000000000 ) ) ;
#26023=ADVANCED_FACE ( 'NONE', ( #16444 ), #30954, .T. ) ;
#26039=CARTESIAN_POINT ( 'NONE',  ( 92.60208470531341618, 155.0000000000000000, 0.000000000000000000 ) ) ;
#26052=DIRECTION ( 'NONE',  ( 0.9945218953682747332, 0.000000000000000000, -0.1045284632676402453 ) ) ;
#26056=AXIS2_PLACEMENT_3D ( 'NONE', #5079, #15300, #26194 ) ;
#26063=ORIENTED_EDGE ( 'NONE', *, *, #19558, .T. ) ;
#26066=DIRECTION ( 'NONE',  ( 0.000000000000000000, 0.000000000000000000, -1.000000000000000000 ) ) ;
#26103=ORIENTED_EDGE ( 'NONE', *, *, #18695, .F. ) ;
#26119=DIRECTION ( 'NONE',  ( 0.9945218953682747332, 1.280104479605073142E-17, 0.1045284632676402453 ) ) ;
#26136=ORIENTED_EDGE ( 'NONE', *, *, #15621, .T. ) ;
#26148=EDGE_CURVE ( 'NONE', #17290, #22749, #26842, .T. ) ;
#26156=CARTESIAN_POINT ( 'NONE',  ( 102.4138169258850581, 155.0000000000000000, 0.000000000000000000 ) ) ;
#26194=DIRECTION ( 'NONE',  ( 0.000000000000000000, 0.000000000000000000, -1.000000000000000000 ) ) ;
#26264=CIRCLE ( 'NONE', #8295, 32.00000000000002842 ) ;
#26280=LINE ( 'NONE', #18283, #22705 ) ;
#26306=EDGE_LOOP ( 'NONE', ( #19374, #15780, #12437, #24368 ) ) ;
#26313=VECTOR ( 'NONE', #14007, 1000.000000000000000 ) ;
#26317=LINE ( 'NONE', #2659, #11833 ) ;
#26344=VERTEX_POINT ( 'NONE', #18840 ) ;
#26384=ADVANCED_FACE ( 'NONE', ( #9463 ), #19850, .T. ) ;
#26392=PRESENTATION_STYLE_ASSIGNMENT (( #16000 ) ) ;
#26437=EDGE_CURVE ( 'NONE', #14059, #4327, #27687, .T. ) ;
#26453=VERTEX_POINT ( 'NONE', #6906 ) ;
#26456=CARTESIAN_POINT ( 'NONE',  ( 95.70416941062676131, 155.0000000000000000, 32.00000000000005684 ) ) ;
#26466=DIRECTION ( 'NONE',  ( 1.000000000000000000, -0.000000000000000000, -0.000000000000000000 ) ) ;
#26467=CONICAL_SURFACE ( 'NONE', #32443, 32.10452846326764131, 1.466076571675242413 ) ;
#26476=CYLINDRICAL_SURFACE ( 'NONE', #21625, 31.00000000000000000 ) ;
#26489=ORIENTED_EDGE ( 'NONE', *, *, #27856, .F. ) ;
#26517=DIRECTION ( 'NONE',  ( 1.000000000000000000, -0.000000000000000000, -0.000000000000000000 ) ) ;
#26533=CARTESIAN_POINT ( 'NONE',  ( 100.3117322205716420, 155.0000000000000000, -12.10452846326767684 ) ) ;
#26582=CIRCLE ( 'NONE', #17351, 12.10452846326765020 ) ;
#26622=VECTOR ( 'NONE', #31530, 999.9999999999998863 ) ;
#26631=CONICAL_SURFACE ( 'NONE', #23426, 32.10452846326764131, 1.466076571675242413 ) ;
#26664=VERTEX_POINT ( 'NONE', #23087 ) ;
#26709=DIRECTION ( 'NONE',  ( 0.000000000000000000, 0.000000000000000000, -1.000000000000000000 ) ) ;
#26776=DIRECTION ( 'NONE',  ( 1.000000000000000000, -0.000000000000000000, -0.000000000000000000 ) ) ;
#26793=ORIENTED_EDGE ( 'NONE', *, *, #7429, .F. ) ;
#26815=LINE ( 'NONE', #3479, #7034 ) ;
#26828=CARTESIAN_POINT ( 'NONE',  ( 93.60208470531338776, 155.0000000000000000, -12.00000000000001066 ) ) ;
#26837=VECTOR ( 'NONE', #12137, 1000.000000000000000 ) ;
#26839=AXIS2_PLACEMENT_3D ( 'NONE', #8236, #11459, #31570 ) ;
#26842=LINE ( 'NONE', #7964, #4283 ) ;
#26864=EDGE_CURVE ( 'NONE', #6991, #9110, #8004, .T. ) ;
#26874=ORIENTED_EDGE ( 'NONE', *, *, #31076, .T. ) ;
#26879=EDGE_CURVE ( 'NONE', #82, #23779, #5816, .T. ) ;
#26886=CARTESIAN_POINT ( 'NONE',  ( 94.70964751525852421, 155.0000000000000000, 0.000000000000000000 ) ) ;
#26891=FILL_AREA_STYLE_COLOUR ( '', #12194 ) ;
#26893=DIRECTION ( 'NONE',  ( -1.000000000000000000, 0.000000000000000000, 0.000000000000000000 ) ) ;
#26926=VERTEX_POINT ( 'NONE', #18805 ) ;
#26931=ORIENTED_EDGE ( 'NONE', *, *, #23649, .F. ) ;
#26950=ORIENTED_EDGE ( 'NONE', *, *, #14769, .T. ) ;
#26954=CARTESIAN_POINT ( 'NONE',  ( 89.50000000000002842, 155.0000000000000000, -32.00000000000002842 ) ) ;
#27053=FACE_OUTER_BOUND ( 'NONE', #23698, .T. ) ;
#27058=FACE_OUTER_BOUND ( 'NONE', #27541, .T. ) ;
#27088=DIRECTION ( 'NONE',  ( 1.000000000000000000, -0.000000000000000000, -0.000000000000000000 ) ) ;
#27125=VERTEX_POINT ( 'NONE', #8106 ) ;
#27153=AXIS2_PLACEMENT_3D ( 'NONE', #10835, #3154, #23609 ) ;
#27157=CARTESIAN_POINT ( 'NONE',  ( 92.60208470531341618, 155.0000000000000000, 13.00000000000002487 ) ) ;
#27182=ADVANCED_FACE ( 'NONE', ( #31277 ), #26476, .F. ) ;
#27184=ORIENTED_EDGE ( 'NONE', *, *, #25408, .T. ) ;
#27194=LINE ( 'NONE', #3188, #5559 ) ;
#27240=EDGE_CURVE ( 'NONE', #1694, #2760, #26317, .T. ) ;
#27254=ORIENTED_EDGE ( 'NONE', *, *, #12033, .T. ) ;
#27296=CIRCLE ( 'NONE', #2284, 12.10452846326767684 ) ;
#27324=AXIS2_PLACEMENT_3D ( 'NONE', #24210, #21152, #29487 ) ;
#27330=EDGE_LOOP ( 'NONE', ( #24868, #20448, #29891, #12889 ) ) ;
#27339=ORIENTED_EDGE ( 'NONE', *, *, #18291, .T. ) ;
#27374=ORIENTED_EDGE ( 'NONE', *, *, #25562, .F. ) ;
#27382=CONICAL_SURFACE ( 'NONE', #8880, 32.00000000000002842, 1.466076571675244411 ) ;
#27406=FACE_OUTER_BOUND ( 'NONE', #33248, .T. ) ;
#27422=EDGE_CURVE ( 'NONE', #16362, #17208, #19439, .T. ) ;
#27440=DIRECTION ( 'NONE',  ( 0.000000000000000000, 0.000000000000000000, -1.000000000000000000 ) ) ;
#27484=CARTESIAN_POINT ( 'NONE',  ( 95.70416941062676131, 155.0000000000000000, -32.00000000000005684 ) ) ;
#27506=EDGE_CURVE ( 'NONE', #16034, #26664, #24432, .T. ) ;
#27513=EDGE_CURVE ( 'NONE', #11140, #17374, #25990, .T. ) ;
#27541=EDGE_LOOP ( 'NONE', ( #21205, #21833, #5144, #33135 ) ) ;
#27552=ORIENTED_EDGE ( 'NONE', *, *, #18695, .T. ) ;
#27585=CARTESIAN_POINT ( 'NONE',  ( 98.19869130599479945, 155.0000000000000000, 0.000000000000000000 ) ) ;
#27603=FILL_AREA_STYLE ('',( #17215 ) ) ;
#27605=VECTOR ( 'NONE', #19316, 1000.000000000000000 ) ;
#27618=ORIENTED_EDGE ( 'NONE', *, *, #2040, .F. ) ;
#27621=LINE ( 'NONE', #4291, #3446 ) ;
#27649=CIRCLE ( 'NONE', #5878, 11.99999999999998224 ) ;
#27664=ADVANCED_FACE ( 'NONE', ( #25440 ), #12933, .T. ) ;
#27673=EDGE_CURVE ( 'NONE', #23405, #6991, #9597, .T. ) ;
#27687=LINE ( 'NONE', #29914, #29750 ) ;
#27694=AXIS2_PLACEMENT_3D ( 'NONE', #33286, #26776, #18622 ) ;
#27733=CARTESIAN_POINT ( 'NONE',  ( 98.19869130599479945, 155.0000000000000000, -32.10452846326769816 ) ) ;
#27752=ORIENTED_EDGE ( 'NONE', *, *, #23038, .T. ) ;
#27778=CIRCLE ( 'NONE', #21264, 32.00000000000002842 ) ;
#27830=EDGE_LOOP ( 'NONE', ( #24109, #23949, #27752, #10729 ) ) ;
#27853=AXIS2_PLACEMENT_3D ( 'NONE', #1046, #19268, #18606 ) ;
#27856=EDGE_CURVE ( 'NONE', #18054, #24364, #26280, .T. ) ;
#27882=EDGE_LOOP ( 'NONE', ( #5595, #27552, #12993, #10105 ) ) ;
#27889=EDGE_CURVE ( 'NONE', #23288, #32773, #8054, .T. ) ;
#27894=AXIS2_PLACEMENT_3D ( 'NONE', #134, #15468, #12907 ) ;
#27928=PRODUCT_DEFINITION_SHAPE ( 'NONE', 'NONE',  #32279 ) ;
#27933=ORIENTED_EDGE ( 'NONE', *, *, #31812, .F. ) ;
#27934=AXIS2_PLACEMENT_3D ( 'NONE', #24048, #3778, #32217 ) ;
#27941=ORIENTED_EDGE ( 'NONE', *, *, #30201, .F. ) ;
#28007=ORIENTED_EDGE ( 'NONE', *, *, #26879, .T. ) ;
#28061=CARTESIAN_POINT ( 'NONE',  ( 104.9083388212530537, 155.0000000000000000, 0.000000000000000000 ) ) ;
#28067=VERTEX_POINT ( 'NONE', #885 ) ;
#28081=CARTESIAN_POINT ( 'NONE',  ( 110.1179863365115636, 155.0000000000000000, 32.10452846326764131 ) ) ;
#28128=ADVANCED_FACE ( 'NONE', ( #9052 ), #20568, .F. ) ;
#28132=DIRECTION ( 'NONE',  ( -0.1045284632676468234, 0.000000000000000000, 0.9945218953682740670 ) ) ;
#28183=CARTESIAN_POINT ( 'NONE',  ( 90.49452189536829394, 155.0000000000000000, 0.000000000000000000 ) ) ;
#28197=ORIENTED_EDGE ( 'NONE', *, *, #17799, .T. ) ;
#28210=DIRECTION ( 'NONE',  ( 0.000000000000000000, 0.000000000000000000, -1.000000000000000000 ) ) ;
#28226=DIRECTION ( 'NONE',  ( 1.000000000000000000, -0.000000000000000000, -0.000000000000000000 ) ) ;
#28238=ORIENTED_EDGE ( 'NONE', *, *, #10027, .T. ) ;
#28253=DIRECTION ( 'NONE',  ( 0.000000000000000000, 0.000000000000000000, -1.000000000000000000 ) ) ;
#28272=AXIS2_PLACEMENT_3D ( 'NONE', #15520, #2074, #5295 ) ;
#28276=FACE_OUTER_BOUND ( 'NONE', #18420, .T. ) ;
#28297=( NAMED_UNIT ( * ) SI_UNIT ( $, .STERADIAN. ) SOLID_ANGLE_UNIT ( ) );
#28298=EDGE_CURVE ( 'NONE', #25373, #5220, #12119, .T. ) ;
#28344=FACE_OUTER_BOUND ( 'NONE', #10145, .T. ) ;
#28369=ORIENTED_EDGE ( 'NONE', *, *, #25212, .F. ) ;
#28384=DIRECTION ( 'NONE',  ( 0.000000000000000000, 0.000000000000000000, -1.000000000000000000 ) ) ;
#28412=EDGE_LOOP ( 'NONE', ( #9536, #15855, #8209, #14308 ) ) ;
#28415=CARTESIAN_POINT ( 'NONE',  ( 105.0134430565187387, 155.0000000000000000, 31.00000000000000000 ) ) ;
#28451=DIRECTION ( 'NONE',  ( 1.000000000000000000, -0.000000000000000000, -0.000000000000000000 ) ) ;
#28496=ADVANCED_FACE ( 'NONE', ( #25397 ), #15111, .F. ) ;
#28499=ORIENTED_EDGE ( 'NONE', *, *, #14980, .F. ) ;
#28516=DIRECTION ( 'NONE',  ( 1.000000000000000000, -0.000000000000000000, -0.000000000000000000 ) ) ;
#28569=EDGE_CURVE ( 'NONE', #2210, #8132, #12417, .T. ) ;
#28595=DIRECTION ( 'NONE',  ( -1.000000000000000000, 0.000000000000000000, 0.000000000000000000 ) ) ;
#28614=CARTESIAN_POINT ( 'NONE',  ( 93.60208470531338776, 155.0000000000000000, 0.000000000000000000 ) ) ;
#28649=EDGE_LOOP ( 'NONE', ( #25412, #31815, #15072, #23728 ) ) ;
#28684=ORIENTED_EDGE ( 'NONE', *, *, #7715, .F. ) ;
#28690=ORIENTED_EDGE ( 'NONE', *, *, #29071, .F. ) ;
#28692=ADVANCED_FACE ( 'NONE', ( #23521 ), #12392, .T. ) ;
#28695=EDGE_LOOP ( 'NONE', ( #30240, #18013, #6645, #17404 ) ) ;
#28724=DIRECTION ( 'NONE',  ( 1.000000000000000000, -0.000000000000000000, -0.000000000000000000 ) ) ;
#28740=DIRECTION ( 'NONE',  ( 0.1045284632676459352, 0.000000000000000000, -0.9945218953682740670 ) ) ;
#28742=UNCERTAINTY_MEASURE_WITH_UNIT (LENGTH_MEASURE( 1.000000000000000082E-05 ), #21117, 'distance_accuracy_value', 'NONE');
#28756=CIRCLE ( 'NONE', #4253, 31.00000000000000000 ) ;
#28781=CARTESIAN_POINT ( 'NONE',  ( 92.60208470531341618, 155.0000000000000000, 0.000000000000000000 ) ) ;
#28791=FACE_OUTER_BOUND ( 'NONE', #18931, .T. ) ;
#28815=UNCERTAINTY_MEASURE_WITH_UNIT (LENGTH_MEASURE( 1.000000000000000082E-05 ), #20951, 'distance_accuracy_value', 'NONE');
#28824=CIRCLE ( 'NONE', #16698, 11.99999999999998224 ) ;
#28864=CARTESIAN_POINT ( 'NONE',  ( 101.3062541159399075, 155.0000000000000000, 0.000000000000000000 ) ) ;
#28909=CARTESIAN_POINT ( 'NONE',  ( 92.70168066101555837, 155.0000000000000000, 0.000000000000000000 ) ) ;
#28932=CARTESIAN_POINT ( 'NONE',  ( 91.60208470531341618, 155.0000000000000000, 0.000000000000000000 ) ) ;
#28950=SURFACE_STYLE_FILL_AREA ( #330 ) ;
#29002=DIRECTION ( 'NONE',  ( 0.1045284632676459352, 1.217938055844715641E-16, 0.9945218953682740670 ) ) ;
#29013=VECTOR ( 'NONE', #21683, 1000.000000000000000 ) ;
#29020=CARTESIAN_POINT ( 'NONE',  ( 91.60208470531341618, 155.0000000000000000, 12.00000000000001066 ) ) ;
#29022=ORIENTED_EDGE ( 'NONE', *, *, #11053, .F. ) ;
#29052=CARTESIAN_POINT ( 'NONE',  ( 102.4138169258850581, 155.0000000000000000, 0.000000000000000000 ) ) ;
#29067=EDGE_CURVE ( 'NONE', #19123, #4327, #11737, .T. ) ;
#29070=DIRECTION ( 'NONE',  ( 0.000000000000000000, 0.000000000000000000, -1.000000000000000000 ) ) ;
#29071=EDGE_CURVE ( 'NONE', #32773, #9926, #16846, .T. ) ;
#29080=DIRECTION ( 'NONE',  ( 0.000000000000000000, 0.000000000000000000, -1.000000000000000000 ) ) ;
#29137=ORIENTED_EDGE ( 'NONE', *, *, #27513, .T. ) ;
#29139=ADVANCED_FACE ( 'NONE', ( #27406 ), #22780, .T. ) ;
#29148=VERTEX_POINT ( 'NONE', #28081 ) ;
#29155=FACE_OUTER_BOUND ( 'NONE', #4431, .T. ) ;
#29169=CARTESIAN_POINT ( 'NONE',  ( 107.0104235265664556, 155.0000000000000000, 0.000000000000000000 ) ) ;
#29179=FACE_OUTER_BOUND ( 'NONE', #1617, .T. ) ;
#29184=DIRECTION ( 'NONE',  ( -0.9945218953682772867, 1.280104479604772081E-17, -0.1045284632676156678 ) ) ;
#29189=CIRCLE ( 'NONE', #3621, 32.10452846326766974 ) ;
#29197=EDGE_LOOP ( 'NONE', ( #26489, #10631, #23079, #28197 ) ) ;
#29217=VERTEX_POINT ( 'NONE', #15134 ) ;
#29230=VECTOR ( 'NONE', #24880, 1000.000000000000000 ) ;
#29258=AXIS2_PLACEMENT_3D ( 'NONE', #25119, #20981, #4511 ) ;
#29277=DIRECTION ( 'NONE',  ( 1.000000000000000000, -0.000000000000000000, -0.000000000000000000 ) ) ;
#29283=CARTESIAN_POINT ( 'NONE',  ( 111.1125082318798007, 155.0000000000000000, 32.00000000000002842 ) ) ;
#29307=AXIS2_PLACEMENT_3D ( 'NONE', #22029, #11804, #3627 ) ;
#29316=EDGE_LOOP ( 'NONE', ( #2963, #3002, #25717, #3619 ) ) ;
#29341=DIRECTION ( 'NONE',  ( 0.000000000000000000, 0.000000000000000000, -1.000000000000000000 ) ) ;
#29437=CARTESIAN_POINT ( 'NONE',  ( 108.1100194822685836, 155.0000000000000000, -13.00000000000003908 ) ) ;
#29447=DIRECTION ( 'NONE',  ( -0.9945218953682772867, 0.000000000000000000, 0.1045284632676156678 ) ) ;
#29453=AXIS2_PLACEMENT_3D ( 'NONE', #22003, #31721, #16716 ) ;
#29468=ORIENTED_EDGE ( 'NONE', *, *, #24157, .F. ) ;
#29487=DIRECTION ( 'NONE',  ( 0.000000000000000000, 0.000000000000000000, -1.000000000000000000 ) ) ;
#29514=ORIENTED_EDGE ( 'NONE', *, *, #6376, .T. ) ;
#29520=ORIENTED_EDGE ( 'NONE', *, *, #16888, .F. ) ;
#29521=AXIS2_PLACEMENT_3D ( 'NONE', #12210, #28226, #11582 ) ;
#29530=VERTEX_POINT ( 'NONE', #8971 ) ;
#29532=VECTOR ( 'NONE', #17186, 1000.000000000000000 ) ;
#29543=CONICAL_SURFACE ( 'NONE', #6715, 32.00000000000000000, 0.1047197551197278087 ) ;
#29550=EDGE_CURVE ( 'NONE', #24364, #22995, #2090, .T. ) ;
#29559=CARTESIAN_POINT ( 'NONE',  ( 94.70964751525852421, 155.0000000000000000, 32.10452846326766974 ) ) ;
#29565=AXIS2_PLACEMENT_3D ( 'NONE', #17260, #32756, #10117 ) ;
#29586=CARTESIAN_POINT ( 'NONE',  ( 95.59906517536109050, 155.0000000000000000, 0.000000000000000000 ) ) ;
#29614=DIRECTION ( 'NONE',  ( 1.000000000000000000, -0.000000000000000000, -0.000000000000000000 ) ) ;
#29620=ORIENTED_EDGE ( 'NONE', *, *, #21976, .F. ) ;
#29654=EDGE_LOOP ( 'NONE', ( #12777, #21518, #1161, #3903 ) ) ;
#29678=DIRECTION ( 'NONE',  ( 1.000000000000000000, -0.000000000000000000, -0.000000000000000000 ) ) ;
#29688=ORIENTED_EDGE ( 'NONE', *, *, #4540, .T. ) ;
#29705=CARTESIAN_POINT ( 'NONE',  ( 103.4083388212532810, 155.0000000000000000, 0.000000000000000000 ) ) ;
#29716=DIRECTION ( 'NONE',  ( 0.000000000000000000, 0.000000000000000000, -1.000000000000000000 ) ) ;
#29736=ORIENTED_EDGE ( 'NONE', *, *, #27889, .T. ) ;
#29750=VECTOR ( 'NONE', #24970, 1000.000000000000000 ) ;
#29795=AXIS2_PLACEMENT_3D ( 'NONE', #31782, #18835, #4006 ) ;
#29851=AXIS2_PLACEMENT_3D ( 'NONE', #28061, #33513, #26020 ) ;
#29891=ORIENTED_EDGE ( 'NONE', *, *, #4540, .F. ) ;
#29914=CARTESIAN_POINT ( 'NONE',  ( 92.60208470531341618, 155.0000000000000000, 31.00000000000000000 ) ) ;
#29920=ADVANCED_FACE ( 'NONE', ( #2495 ), #10822, .T. ) ;
#29925=EDGE_CURVE ( 'NONE', #17208, #16362, #11906, .T. ) ;
#29946=ORIENTED_EDGE ( 'NONE', *, *, #8334, .F. ) ;
#29956=( NAMED_UNIT ( * ) SI_UNIT ( $, .STERADIAN. ) SOLID_ANGLE_UNIT ( ) );
#29977=VECTOR ( 'NONE', #23471, 1000.000000000000000 ) ;
#29996=EDGE_LOOP ( 'NONE', ( #27618, #27941, #26136, #17378 ) ) ;
#30014=CARTESIAN_POINT ( 'NONE',  ( 90.49452189536829394, 155.0000000000000000, 32.10452846326766974 ) ) ;
#30021=CARTESIAN_POINT ( 'NONE',  ( 109.0104235265664272, 155.0000000000000000, 11.99999999999998224 ) ) ;
#30025=CARTESIAN_POINT ( 'NONE',  ( 99.30625411593993590, 155.0000000000000000, 0.000000000000000000 ) ) ;
#30031=DIRECTION ( 'NONE',  ( 1.000000000000000000, -0.000000000000000000, -0.000000000000000000 ) ) ;
#30075=CIRCLE ( 'NONE', #7226, 32.00000000000005684 ) ;
#30120=FACE_OUTER_BOUND ( 'NONE', #28649, .T. ) ;
#30121=VECTOR ( 'NONE', #13995, 999.9999999999998863 ) ;
#30130=CONICAL_SURFACE ( 'NONE', #19233, 32.10452846326769816, 1.466076571675243079 ) ;
#30199=ORIENTED_EDGE ( 'NONE', *, *, #9062, .T. ) ;
#30201=EDGE_CURVE ( 'NONE', #4805, #21429, #26582, .T. ) ;
#30215=DIRECTION ( 'NONE',  ( 1.000000000000000000, -0.000000000000000000, -0.000000000000000000 ) ) ;
#30221=DIRECTION ( 'NONE',  ( 0.000000000000000000, 0.000000000000000000, 1.000000000000000000 ) ) ;
#30240=ORIENTED_EDGE ( 'NONE', *, *, #27240, .F. ) ;
#30255=CARTESIAN_POINT ( 'NONE',  ( 111.1125082318798007, 155.0000000000000000, -32.00000000000002842 ) ) ;
#30268=CYLINDRICAL_SURFACE ( 'NONE', #29521, 12.10452846326763598 ) ;
#30287=DIRECTION ( 'NONE',  ( 0.000000000000000000, 0.000000000000000000, 1.000000000000000000 ) ) ;
#30306=DIRECTION ( 'NONE',  ( 1.000000000000000000, -0.000000000000000000, -0.000000000000000000 ) ) ;
#30346=DIRECTION ( 'NONE',  ( 0.000000000000000000, 0.000000000000000000, 1.000000000000000000 ) ) ;
#30381=CONICAL_SURFACE ( 'NONE', #24394, 31.00000000000000000, 1.466076571675244411 ) ;
#30448=CYLINDRICAL_SURFACE ( 'NONE', #20534, 13.00000000000002487 ) ;
#30463=DIRECTION ( 'NONE',  ( 1.000000000000000000, -0.000000000000000000, -0.000000000000000000 ) ) ;
#30491=ORIENTED_EDGE ( 'NONE', *, *, #16249, .T. ) ;
#30510=CONICAL_SURFACE ( 'NONE', #15820, 32.00000000000002842, 0.1047197551196217685 ) ;
#30513=CARTESIAN_POINT ( 'NONE',  ( 108.0049454219347354, 155.0000000000000000, -12.10452846326765020 ) ) ;
#30577=EDGE_CURVE ( 'NONE', #21804, #15528, #5281, .T. ) ;
#30616=FACE_OUTER_BOUND ( 'NONE', #16890, .T. ) ;
#30619=ORIENTED_EDGE ( 'NONE', *, *, #11053, .T. ) ;
#30663=CARTESIAN_POINT ( 'NONE',  ( 104.9083388212530537, 155.0000000000000000, -32.00000000000000000 ) ) ;
#30672=STYLED_ITEM ( 'NONE', ( #22502 ), #11828 ) ;
#30702=EDGE_LOOP ( 'NONE', ( #10517, #10755, #30619, #15923 ) ) ;
#30714=( GEOMETRIC_REPRESENTATION_CONTEXT ( 3 ) GLOBAL_UNCERTAINTY_ASSIGNED_CONTEXT ( ( #28815 ) ) GLOBAL_UNIT_ASSIGNED_CONTEXT ( ( #20951, #21605, #174 ) ) REPRESENTATION_CONTEXT ( 'NONE', 'WORKASPACE' ) );
#30715=LINE ( 'NONE', #1576, #26837 ) ;
#30747=CARTESIAN_POINT ( 'NONE',  ( 104.9083388212530537, 155.0000000000000000, 0.000000000000000000 ) ) ;
#30768=ADVANCED_FACE ( 'NONE', ( #16916 ), #6403, .F. ) ;
#30770=FACE_OUTER_BOUND ( 'NONE', #16525, .T. ) ;
#30787=ORIENTED_EDGE ( 'NONE', *, *, #1411, .T. ) ;
#30793=EDGE_LOOP ( 'NONE', ( #2879, #22316, #3805, #23750 ) ) ;
#30798=EDGE_CURVE ( 'NONE', #33389, #31608, #33101, .T. ) ;
#30802=VERTEX_POINT ( 'NONE', #22365 ) ;
#30820=DIRECTION ( 'NONE',  ( 0.000000000000000000, 0.000000000000000000, -1.000000000000000000 ) ) ;
#30857=AXIS2_PLACEMENT_3D ( 'NONE', #22986, #2209, #22822 ) ;
#30878=EDGE_LOOP ( 'NONE', ( #32665, #24621, #7242, #9120 ) ) ;
#30916=AXIS2_PLACEMENT_3D ( 'NONE', #29169, #6507, #16378 ) ;
#30924=CARTESIAN_POINT ( 'NONE',  ( 92.60208470531341618, 155.0000000000000000, -32.00000000000001421 ) ) ;
#30954=CONICAL_SURFACE ( 'NONE', #20614, 32.00000000000002842, 0.1047197551196784177 ) ;
#30984=CARTESIAN_POINT ( 'NONE',  ( 92.60208470531341618, 155.0000000000000000, -31.00000000000000000 ) ) ;
#31009=DIRECTION ( 'NONE',  ( 0.000000000000000000, 0.000000000000000000, -1.000000000000000000 ) ) ;
#31014=DIRECTION ( 'NONE',  ( 0.000000000000000000, 0.000000000000000000, -1.000000000000000000 ) ) ;
#31021=DIRECTION ( 'NONE',  ( -1.000000000000000000, 0.000000000000000000, 0.000000000000000000 ) ) ;
#31051=EDGE_LOOP ( 'NONE', ( #11246, #8697, #21347, #15411 ) ) ;
#31075=CYLINDRICAL_SURFACE ( 'NONE', #4205, 12.10452846326765020 ) ;
#31076=EDGE_CURVE ( 'NONE', #21262, #9926, #24330, .T. ) ;
#31084=ORIENTED_EDGE ( 'NONE', *, *, #29071, .T. ) ;
#31102=CYLINDRICAL_SURFACE ( 'NONE', #14073, 31.00000000000000000 ) ;
#31136=ORIENTED_EDGE ( 'NONE', *, *, #622, .T. ) ;
#31154=DIRECTION ( 'NONE',  ( 1.000000000000000000, -0.000000000000000000, -0.000000000000000000 ) ) ;
#31162=DIRECTION ( 'NONE',  ( 0.1045284632676472814, 1.217938055844715641E-16, 0.9945218953682740670 ) ) ;
#31187=CIRCLE ( 'NONE', #5088, 11.99999999999998224 ) ;
#31239=DIRECTION ( 'NONE',  ( 0.9945218953682747332, 1.280104479605073142E-17, 0.1045284632676402453 ) ) ;
#31252=DIRECTION ( 'NONE',  ( 0.000000000000000000, 0.000000000000000000, -1.000000000000000000 ) ) ;
#31257=ADVANCED_FACE ( 'NONE', ( #27058 ), #26467, .T. ) ;
#31277=FACE_OUTER_BOUND ( 'NONE', #4500, .T. ) ;
#31297=ORIENTED_EDGE ( 'NONE', *, *, #978, .T. ) ;
#31313=DIRECTION ( 'NONE',  ( 0.1045284632676479336, 1.217938055844715641E-16, 0.9945218953682739560 ) ) ;
#31344=DIRECTION ( 'NONE',  ( 1.000000000000000000, -0.000000000000000000, -0.000000000000000000 ) ) ;
#31377=DIRECTION ( 'NONE',  ( 1.000000000000000000, -0.000000000000000000, -0.000000000000000000 ) ) ;
#31380=EDGE_CURVE ( 'NONE', #889, #1694, #25941, .T. ) ;
#31391=DIRECTION ( 'NONE',  ( 1.000000000000000000, -0.000000000000000000, -0.000000000000000000 ) ) ;
#31405=DIRECTION ( 'NONE',  ( 0.000000000000000000, 0.000000000000000000, -1.000000000000000000 ) ) ;
#31411=CONICAL_SURFACE ( 'NONE', #30857, 32.00000000000000000, 0.1047197551197016768 ) ;
#31422=ORIENTED_EDGE ( 'NONE', *, *, #15438, .F. ) ;
#31442=DIRECTION ( 'NONE',  ( 1.000000000000000000, -0.000000000000000000, -0.000000000000000000 ) ) ;
#31474=CARTESIAN_POINT ( 'NONE',  ( 92.60756280994512224, 155.0000000000000000, 12.10452846326762177 ) ) ;
#31501=VERTEX_POINT ( 'NONE', #9852 ) ;
#31524=AXIS2_PLACEMENT_3D ( 'NONE', #3440, #8234, #31405 ) ;
#31530=DIRECTION ( 'NONE',  ( -0.9945218953682777308, 0.000000000000000000, 0.1045284632676128089 ) ) ;
#31570=DIRECTION ( 'NONE',  ( 0.000000000000000000, 0.000000000000000000, -1.000000000000000000 ) ) ;
#31583=VERTEX_POINT ( 'NONE', #31474 ) ;
#31607=DIRECTION ( 'NONE',  ( 1.000000000000000000, -0.000000000000000000, -0.000000000000000000 ) ) ;
#31608=VERTEX_POINT ( 'NONE', #28415 ) ;
#31626=AXIS2_PLACEMENT_3D ( 'NONE', #2186, #2357, #28253 ) ;
#31657=CIRCLE ( 'NONE', #23494, 12.10452846326765020 ) ;
#31663=DIRECTION ( 'NONE',  ( 0.000000000000000000, 0.000000000000000000, -1.000000000000000000 ) ) ;
#31700=EDGE_LOOP ( 'NONE', ( #9494, #8913, #28684, #32038 ) ) ;
#31704=CIRCLE ( 'NONE', #17007, 12.10452846326767684 ) ;
#31720=DIRECTION ( 'NONE',  ( 0.9945218953682777308, 0.000000000000000000, -0.1045284632676113518 ) ) ;
#31721=DIRECTION ( 'NONE',  ( 1.000000000000000000, -0.000000000000000000, -0.000000000000000000 ) ) ;
#31737=CARTESIAN_POINT ( 'NONE',  ( 93.60208470531338776, 155.0000000000000000, 0.000000000000000000 ) ) ;
#31782=CARTESIAN_POINT ( 'NONE',  ( 107.0104235265664556, 155.0000000000000000, 0.000000000000000000 ) ) ;
#31792=AXIS2_PLACEMENT_3D ( 'NONE', #20242, #28595, #20421 ) ;
#31801=FACE_OUTER_BOUND ( 'NONE', #25627, .T. ) ;
#31812=EDGE_CURVE ( 'NONE', #28067, #26664, #715, .T. ) ;
#31815=ORIENTED_EDGE ( 'NONE', *, *, #26437, .T. ) ;
#31819=EDGE_CURVE ( 'NONE', #22749, #15528, #20579, .T. ) ;
#31822=CARTESIAN_POINT ( 'NONE',  ( 105.0134430565187387, 155.0000000000000000, 0.000000000000000000 ) ) ;
#31845=EDGE_CURVE ( 'NONE', #25373, #20010, #15933, .T. ) ;
#31850=CARTESIAN_POINT ( 'NONE',  ( 105.0134430565187387, 155.0000000000000000, 0.000000000000000000 ) ) ;
#31884=DIRECTION ( 'NONE',  ( 0.000000000000000000, 0.000000000000000000, -1.000000000000000000 ) ) ;
#31895=DIRECTION ( 'NONE',  ( 0.000000000000000000, 0.000000000000000000, 1.000000000000000000 ) ) ;
#31941=FACE_OUTER_BOUND ( 'NONE', #27330, .T. ) ;
#31950=CARTESIAN_POINT ( 'NONE',  ( 103.4083388212532810, 155.0000000000000000, 0.000000000000000000 ) ) ;
#31968=AXIS2_PLACEMENT_3D ( 'NONE', #3881, #9502, #30287 ) ;
#31985=ORIENTED_EDGE ( 'NONE', *, *, #17471, .T. ) ;
#32001=CARTESIAN_POINT ( 'NONE',  ( 111.1125082318798007, 155.0000000000000000, 0.000000000000000000 ) ) ;
#32034=ORIENTED_EDGE ( 'NONE', *, *, #12448, .T. ) ;
#32038=ORIENTED_EDGE ( 'NONE', *, *, #32224, .F. ) ;
#32046=CARTESIAN_POINT ( 'NONE',  ( 89.50000000000002842, 155.0000000000000000, 0.000000000000000000 ) ) ;
#32048=DIRECTION ( 'NONE',  ( 1.000000000000000000, -0.000000000000000000, -0.000000000000000000 ) ) ;
#32054=ADVANCED_FACE ( 'NONE', ( #12624 ), #9422, .T. ) ;
#32155=FACE_OUTER_BOUND ( 'NONE', #15023, .T. ) ;
#32198=LINE ( 'NONE', #21980, #22522 ) ;
#32217=DIRECTION ( 'NONE',  ( 0.000000000000000000, 0.000000000000000000, -1.000000000000000000 ) ) ;
#32224=EDGE_CURVE ( 'NONE', #9110, #10473, #849, .T. ) ;
#32231=ORIENTED_EDGE ( 'NONE', *, *, #15768, .T. ) ;
#32241=ORIENTED_EDGE ( 'NONE', *, *, #32838, .F. ) ;
#32248=AXIS2_PLACEMENT_3D ( 'NONE', #11574, #30306, #9520 ) ;
#32259=CARTESIAN_POINT ( 'NONE',  ( 97.30927364589244632, 155.0000000000000000, 0.000000000000000000 ) ) ;
#32279=PRODUCT_DEFINITION ( 'UNKNOWN', '', #19725, #16570 ) ;
#32306=CARTESIAN_POINT ( 'NONE',  ( 108.0049454219347354, 155.0000000000000000, 0.000000000000000000 ) ) ;
#32320=STYLED_ITEM ( 'NONE', ( #26392 ), #9595 ) ;
#32332=ORIENTED_EDGE ( 'NONE', *, *, #1238, .T. ) ;
#32334=( LENGTH_UNIT ( ) NAMED_UNIT ( * ) SI_UNIT ( .MILLI., .METRE. ) );
#32376=FACE_OUTER_BOUND ( 'NONE', #10487, .T. ) ;
#32398=DIRECTION ( 'NONE',  ( -0.9945218953682687379, 0.000000000000000000, 0.1045284632676965614 ) ) ;
#32405=CARTESIAN_POINT ( 'NONE',  ( 99.30625411593993590, 155.0000000000000000, 12.00000000000001066 ) ) ;
#32423=CARTESIAN_POINT ( 'NONE',  ( 95.70416941062676131, 155.0000000000000000, 0.000000000000000000 ) ) ;
#32443=AXIS2_PLACEMENT_3D ( 'NONE', #11726, #5490, #6613 ) ;
#32447=LINE ( 'NONE', #32620, #22147 ) ;
#32456=EDGE_CURVE ( 'NONE', #23779, #82, #1778, .T. ) ;
#32458=AXIS2_PLACEMENT_3D ( 'NONE', #26886, #29277, #3715 ) ;
#32467=DIRECTION ( 'NONE',  ( 0.000000000000000000, 0.000000000000000000, -1.000000000000000000 ) ) ;
#32504=EDGE_CURVE ( 'NONE', #8132, #3157, #7141, .T. ) ;
#32529=ORIENTED_EDGE ( 'NONE', *, *, #4354, .T. ) ;
#32543=DIRECTION ( 'NONE',  ( 1.000000000000000000, -0.000000000000000000, -0.000000000000000000 ) ) ;
#32554=CIRCLE ( 'NONE', #26056, 11.99999999999998224 ) ;
#32555=DIRECTION ( 'NONE',  ( 0.1045284632676479336, 0.000000000000000000, -0.9945218953682739560 ) ) ;
#32558=ADVANCED_FACE ( 'NONE', ( #17526 ), #20293, .T. ) ;
#32583=ORIENTED_EDGE ( 'NONE', *, *, #4354, .F. ) ;
#32593=VECTOR ( 'NONE', #17258, 999.9999999999998863 ) ;
#32597=DIRECTION ( 'NONE',  ( 0.000000000000000000, 0.000000000000000000, -1.000000000000000000 ) ) ;
#32615=CARTESIAN_POINT ( 'NONE',  ( 101.3062541159399075, 155.0000000000000000, -12.00000000000001066 ) ) ;
#32620=CARTESIAN_POINT ( 'NONE',  ( 94.70964751525852421, 155.0000000000000000, -32.10452846326766974 ) ) ;
#32623=ORIENTED_EDGE ( 'NONE', *, *, #21584, .T. ) ;
#32665=ORIENTED_EDGE ( 'NONE', *, *, #6177, .F. ) ;
#32694=ORIENTED_EDGE ( 'NONE', *, *, #7292, .T. ) ;
#32696=EDGE_CURVE ( 'NONE', #14731, #16034, #13793, .T. ) ;
#32704=FACE_OUTER_BOUND ( 'NONE', #4209, .T. ) ;
#32756=DIRECTION ( 'NONE',  ( 1.000000000000000000, -0.000000000000000000, -0.000000000000000000 ) ) ;
#32757=FACE_OUTER_BOUND ( 'NONE', #1106, .T. ) ;
#32766=ORIENTED_EDGE ( 'NONE', *, *, #23140, .F. ) ;
#32767=LINE ( 'NONE', #17110, #2131 ) ;
#32773=VERTEX_POINT ( 'NONE', #25874 ) ;
#32784=CARTESIAN_POINT ( 'NONE',  ( 92.60208470531341618, 155.0000000000000000, 0.000000000000000000 ) ) ;
#32792=VECTOR ( 'NONE', #9797, 999.9999999999998863 ) ;
#32796=CARTESIAN_POINT ( 'NONE',  ( 107.0104235265664556, 155.0000000000000000, -11.99999999999998224 ) ) ;
#32828=ADVANCED_FACE ( 'NONE', ( #33376 ), #27382, .F. ) ;
#32837=FACE_OUTER_BOUND ( 'NONE', #9399, .T. ) ;
#32838=EDGE_CURVE ( 'NONE', #1694, #889, #195, .T. ) ;
#32868=DIRECTION ( 'NONE',  ( 0.000000000000000000, 0.000000000000000000, -1.000000000000000000 ) ) ;
#32912=DIRECTION ( 'NONE',  ( 0.000000000000000000, 0.000000000000000000, -1.000000000000000000 ) ) ;
#32955=DIRECTION ( 'NONE',  ( 1.000000000000000000, -0.000000000000000000, -0.000000000000000000 ) ) ;
#32956=EDGE_LOOP ( 'NONE', ( #16281, #10029, #14602, #25156 ) ) ;
#32969=VECTOR ( 'NONE', #22373, 1000.000000000000227 ) ;
#32978=EDGE_CURVE ( 'NONE', #23288, #21869, #14972, .T. ) ;
#32988=DIRECTION ( 'NONE',  ( 1.000000000000000000, -0.000000000000000000, -0.000000000000000000 ) ) ;
#32995=VECTOR ( 'NONE', #8522, 1000.000000000000000 ) ;
#33000=CARTESIAN_POINT ( 'NONE',  ( 100.3007760113082156, 155.0000000000000000, -12.10452846326762177 ) ) ;
#33004=CARTESIAN_POINT ( 'NONE',  ( 102.4138169258850581, 155.0000000000000000, -32.10452846326769816 ) ) ;
#33017=AXIS2_PLACEMENT_3D ( 'NONE', #10996, #31607, #8436 ) ;
#33022=DIRECTION ( 'NONE',  ( 1.000000000000000000, -0.000000000000000000, -0.000000000000000000 ) ) ;
#33032=FACE_OUTER_BOUND ( 'NONE', #29197, .T. ) ;
#33077=CARTESIAN_POINT ( 'NONE',  ( 92.60208470531341618, 155.0000000000000000, 0.000000000000000000 ) ) ;
#33086=AXIS2_PLACEMENT_3D ( 'NONE', #189, #5290, #10587 ) ;
#33091=CARTESIAN_POINT ( 'NONE',  ( 108.0049454219347354, 155.0000000000000000, 12.10452846326765020 ) ) ;
#33101=LINE ( 'NONE', #25092, #32593 ) ;
#33103=PRODUCT ( 'High-Force Belleville Spring Washer Pack', 'High-Force Belleville Spring Washer Pack', '', ( #16165 ) ) ;
#33105=AXIS2_PLACEMENT_3D ( 'NONE', #11388, #29614, #26709 ) ;
#33135=ORIENTED_EDGE ( 'NONE', *, *, #179, .F. ) ;
#33187=DIRECTION ( 'NONE',  ( 1.000000000000000000, -0.000000000000000000, -0.000000000000000000 ) ) ;
#33225=VERTEX_POINT ( 'NONE', #21030 ) ;
#33248=EDGE_LOOP ( 'NONE', ( #16069, #32694, #5884, #18222 ) ) ;
#33286=CARTESIAN_POINT ( 'NONE',  ( 99.30625411593993590, 155.0000000000000000, 0.000000000000000000 ) ) ;
#33315=VECTOR ( 'NONE', #24381, 1000.000000000000227 ) ;
#33321=DIRECTION ( 'NONE',  ( 1.000000000000000000, -0.000000000000000000, -0.000000000000000000 ) ) ;
#33355=EDGE_LOOP ( 'NONE', ( #12089, #23947, #6518, #19167 ) ) ;
#33368=CONICAL_SURFACE ( 'NONE', #3977, 12.00000000000001066, 0.1047197551196188681 ) ;
#33376=FACE_OUTER_BOUND ( 'NONE', #25378, .T. ) ;
#33389=VERTEX_POINT ( 'NONE', #7420 ) ;
#33395=AXIS2_PLACEMENT_3D ( 'NONE', #17415, #4466, #1918 ) ;
#33398=CONICAL_SURFACE ( 'NONE', #4550, 31.00000000000000000, 1.466076571675255957 ) ;
#33416=DIRECTION ( 'NONE',  ( -1.000000000000000000, 0.000000000000000000, 0.000000000000000000 ) ) ;
#33460=EDGE_CURVE ( 'NONE', #23779, #2760, #2652, .T. ) ;
#33470=CARTESIAN_POINT ( 'NONE',  ( 93.60208470531338776, 155.0000000000000000, -12.00000000000001066 ) ) ;
#33487=EDGE_CURVE ( 'NONE', #29530, #21262, #17080, .T. ) ;
#33513=DIRECTION ( 'NONE',  ( 1.000000000000000000, -0.000000000000000000, -0.000000000000000000 ) ) ;
#33547=AXIS2_PLACEMENT_3D ( 'NONE', #33077, #24746, #19629 ) ;
#33580=DIRECTION ( 'NONE',  ( 0.000000000000000000, 0.000000000000000000, -1.000000000000000000 ) ) ;
#33620=VECTOR ( 'NONE', #33187, 1000.000000000000000 ) ;
#33622=CARTESIAN_POINT ( 'NONE',  ( 103.3032345859876102, 155.0000000000000000, -31.00000000000000000 ) ) ;
ENDSEC;
END-ISO-10303-21;
